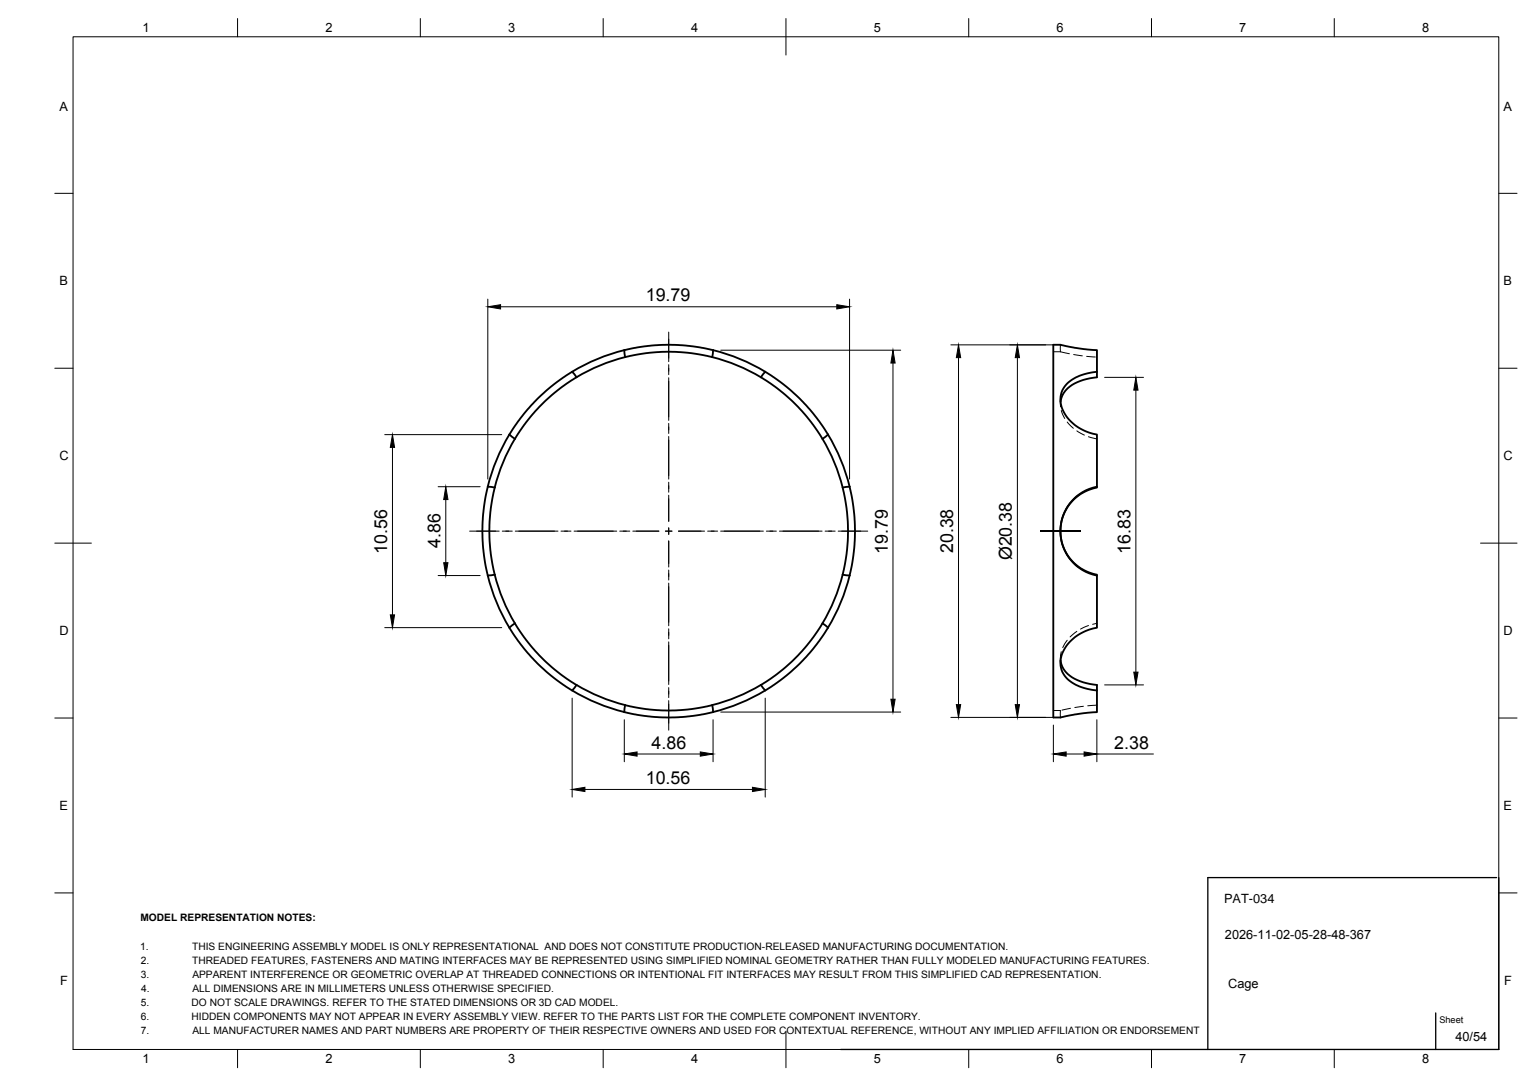
ISO-10303-21;
HEADER;
/* Generated by software containing ST-Developer
 * from STEP Tools, Inc. (www.steptools.com) 
 */

FILE_DESCRIPTION(
/* description */ ('Fatigue rig crank-slider'),
/* implementation_level */ '2;1');

FILE_NAME(
/* name */ 'Cage.step',
/* time_stamp */ '2026-10-28T03:24:50-07:00',
/* author */ (''),
/* organization */ (''),
/* preprocessor_version */ 'ST-DEVELOPER v20.2',
/* originating_system */ 'Autodesk Translation Framework v15.17.0.0',
/* authorisation */ '');

FILE_SCHEMA (('AUTOMOTIVE_DESIGN { 1 0 10303 214 3 1 1 }'));
ENDSEC;

DATA;
#10=MECHANICAL_DESIGN_GEOMETRIC_PRESENTATION_REPRESENTATION('',(#630),#16911);
#451=B_SPLINE_CURVE_WITH_KNOTS('',3,(#15536,#15537,#15538,#15539,#15540,
#15541,#15542,#15543,#15544,#15545,#15546,#15547,#15548,#15549,#15550,#15551,
#15552,#15553,#15554,#15555,#15556,#15557),.UNSPECIFIED.,.F.,.F.,(4,2,2,
2,2,2,2,2,2,2,4),(0.0473477652366656,0.126350602536658,0.189525903804987,
0.252701205073317,0.313298422430275,0.373895639787233,0.434492857144191,
0.495090074501149,0.558265375769478,0.621440677037807,0.7004435143378),
 .UNSPECIFIED.);
#452=B_SPLINE_CURVE_WITH_KNOTS('',3,(#15561,#15562,#15563,#15564,#15565,
#15566,#15567,#15568,#15569,#15570,#15571,#15572,#15573,#15574,#15575,#15576,
#15577,#15578,#15579,#15580,#15581,#15582),.UNSPECIFIED.,.F.,.F.,(4,2,2,
2,2,2,2,2,2,2,4),(0.0464897534940957,0.0852567806515119,0.170513561303024,
0.246687263103517,0.308657850341199,0.370628437578881,0.432599024816563,
0.494569612054245,0.570743313854739,0.656000094506251,0.694767121663666),
 .UNSPECIFIED.);
#453=B_SPLINE_CURVE_WITH_KNOTS('',3,(#15588,#15589,#15590,#15591,#15592,
#15593,#15594,#15595,#15596,#15597,#15598,#15599,#15600,#15601,#15602,#15603,
#15604,#15605,#15606,#15607,#15608,#15609),.UNSPECIFIED.,.F.,.F.,(4,2,2,
2,2,2,2,2,2,2,4),(0.0464897534940957,0.0852567806515118,0.170513561303024,
0.246687263103517,0.308657850341199,0.370628437578881,0.432599024816563,
0.494569612054245,0.570743313854738,0.65600009450625,0.694767121663666),
 .UNSPECIFIED.);
#454=B_SPLINE_CURVE_WITH_KNOTS('',3,(#15613,#15614,#15615,#15616,#15617,
#15618,#15619,#15620,#15621,#15622,#15623,#15624,#15625,#15626,#15627,#15628,
#15629,#15630,#15631,#15632,#15633,#15634),.UNSPECIFIED.,.F.,.F.,(4,2,2,
2,2,2,2,2,2,2,4),(0.0464897534940957,0.0852567806515119,0.170513561303024,
0.246687263103517,0.308657850341199,0.370628437578881,0.432599024816563,
0.494569612054245,0.570743313854739,0.656000094506251,0.694767121663666),
 .UNSPECIFIED.);
#455=B_SPLINE_CURVE_WITH_KNOTS('',3,(#15638,#15639,#15640,#15641,#15642,
#15643,#15644,#15645,#15646,#15647,#15648,#15649),.UNSPECIFIED.,.F.,.F.,
(4,2,2,2,2,4),(0.0464897534940957,0.0852567806515119,0.170513561303024,
0.246687263103517,0.308657850341199,0.370628437578881),.UNSPECIFIED.);
#456=B_SPLINE_CURVE_WITH_KNOTS('',3,(#15654,#15655,#15656,#15657,#15658,
#15659,#15660,#15661,#15662,#15663,#15664,#15665),.UNSPECIFIED.,.F.,.F.,
(4,2,2,2,2,4),(0.370628437578881,0.432599024816563,0.494569612054245,0.570743313854738,
0.65600009450625,0.694767121663666),.UNSPECIFIED.);
#457=B_SPLINE_CURVE_WITH_KNOTS('',3,(#15669,#15670,#15671,#15672,#15673,
#15674,#15675,#15676,#15677,#15678,#15679,#15680,#15681,#15682,#15683,#15684,
#15685,#15686,#15687,#15688,#15689,#15690),.UNSPECIFIED.,.F.,.F.,(4,2,2,
2,2,2,2,2,2,2,4),(0.0464897534940957,0.0852567806515121,0.170513561303024,
0.246687263103518,0.308657850341199,0.370628437578881,0.432599024816563,
0.494569612054245,0.570743313854738,0.65600009450625,0.694767121663666),
 .UNSPECIFIED.);
#458=B_SPLINE_CURVE_WITH_KNOTS('',3,(#15694,#15695,#15696,#15697,#15698,
#15699,#15700,#15701,#15702,#15703,#15704,#15705,#15706,#15707,#15708,#15709,
#15710,#15711,#15712,#15713,#15714,#15715),.UNSPECIFIED.,.F.,.F.,(4,2,2,
2,2,2,2,2,2,2,4),(0.0464897534940957,0.0852567806515119,0.170513561303024,
0.246687263103517,0.308657850341199,0.370628437578881,0.432599024816563,
0.494569612054245,0.570743313854738,0.65600009450625,0.694767121663667),
 .UNSPECIFIED.);
#459=B_SPLINE_CURVE_WITH_KNOTS('',3,(#15719,#15720,#15721,#15722,#15723,
#15724,#15725,#15726,#15727,#15728,#15729,#15730,#15731,#15732,#15733,#15734,
#15735,#15736,#15737,#15738,#15739,#15740),.UNSPECIFIED.,.F.,.F.,(4,2,2,
2,2,2,2,2,2,2,4),(0.0464897534940957,0.0852567806515119,0.170513561303024,
0.246687263103517,0.308657850341199,0.370628437578881,0.432599024816563,
0.494569612054245,0.570743313854738,0.65600009450625,0.694767121663666),
 .UNSPECIFIED.);
#460=B_SPLINE_CURVE_WITH_KNOTS('',3,(#15744,#15745,#15746,#15747,#15748,
#15749,#15750,#15751,#15752,#15753,#15754,#15755,#15756,#15757,#15758,#15759,
#15760,#15761,#15762,#15763,#15764,#15765),.UNSPECIFIED.,.F.,.F.,(4,2,2,
2,2,2,2,2,2,2,4),(0.0464897534940957,0.0852567806515119,0.170513561303024,
0.246687263103517,0.308657850341199,0.370628437578881,0.432599024816563,
0.494569612054245,0.570743313854739,0.656000094506251,0.694767121663667),
 .UNSPECIFIED.);
#461=B_SPLINE_CURVE_WITH_KNOTS('',3,(#15773,#15774,#15775,#15776,#15777,
#15778,#15779,#15780,#15781,#15782,#15783,#15784,#15785,#15786,#15787,#15788,
#15789,#15790,#15791,#15792,#15793,#15794),.UNSPECIFIED.,.F.,.F.,(4,2,2,
2,2,2,2,2,2,2,4),(0.0473477652366656,0.126350602536658,0.189525903804987,
0.252701205073316,0.313298422430274,0.373895639787232,0.434492857144191,
0.495090074501149,0.558265375769478,0.621440677037807,0.7004435143378),
 .UNSPECIFIED.);
#462=B_SPLINE_CURVE_WITH_KNOTS('',3,(#15802,#15803,#15804,#15805,#15806,
#15807,#15808,#15809,#15810,#15811,#15812,#15813,#15814,#15815,#15816,#15817,
#15818,#15819,#15820,#15821,#15822,#15823),.UNSPECIFIED.,.F.,.F.,(4,2,2,
2,2,2,2,2,2,2,4),(0.0473477652366656,0.126350602536658,0.189525903804987,
0.252701205073317,0.313298422430275,0.373895639787233,0.434492857144191,
0.495090074501149,0.558265375769478,0.621440677037807,0.7004435143378),
 .UNSPECIFIED.);
#463=B_SPLINE_CURVE_WITH_KNOTS('',3,(#15832,#15833,#15834,#15835,#15836,
#15837,#15838,#15839,#15840,#15841,#15842,#15843),.UNSPECIFIED.,.F.,.F.,
(4,2,2,2,2,4),(0.0473477652366656,0.126350602536658,0.189525903804987,0.252701205073316,
0.313298422430275,0.373895639787233),.UNSPECIFIED.);
#464=B_SPLINE_CURVE_WITH_KNOTS('',3,(#15845,#15846,#15847,#15848,#15849,
#15850,#15851,#15852,#15853,#15854,#15855,#15856),.UNSPECIFIED.,.F.,.F.,
(4,2,2,2,2,4),(0.373895639787233,0.434492857144191,0.495090074501149,0.558265375769478,
0.621440677037807,0.7004435143378),.UNSPECIFIED.);
#465=B_SPLINE_CURVE_WITH_KNOTS('',3,(#15863,#15864,#15865,#15866,#15867,
#15868,#15869,#15870,#15871,#15872,#15873,#15874,#15875,#15876,#15877,#15878,
#15879,#15880,#15881,#15882,#15883,#15884),.UNSPECIFIED.,.F.,.F.,(4,2,2,
2,2,2,2,2,2,2,4),(0.0473477652366656,0.126350602536658,0.189525903804987,
0.252701205073316,0.313298422430275,0.373895639787233,0.434492857144191,
0.495090074501149,0.558265375769478,0.621440677037807,0.7004435143378),
 .UNSPECIFIED.);
#466=B_SPLINE_CURVE_WITH_KNOTS('',3,(#15892,#15893,#15894,#15895,#15896,
#15897,#15898,#15899,#15900,#15901,#15902,#15903,#15904,#15905,#15906,#15907,
#15908,#15909,#15910,#15911,#15912,#15913),.UNSPECIFIED.,.F.,.F.,(4,2,2,
2,2,2,2,2,2,2,4),(0.0473477652366656,0.126350602536658,0.189525903804987,
0.252701205073317,0.313298422430275,0.373895639787233,0.434492857144191,
0.495090074501149,0.558265375769478,0.621440677037807,0.7004435143378),
 .UNSPECIFIED.);
#467=B_SPLINE_CURVE_WITH_KNOTS('',3,(#15921,#15922,#15923,#15924,#15925,
#15926,#15927,#15928,#15929,#15930,#15931,#15932,#15933,#15934,#15935,#15936,
#15937,#15938,#15939,#15940,#15941,#15942),.UNSPECIFIED.,.F.,.F.,(4,2,2,
2,2,2,2,2,2,2,4),(0.0473477652366656,0.126350602536658,0.189525903804987,
0.252701205073316,0.313298422430275,0.373895639787233,0.434492857144191,
0.495090074501149,0.558265375769478,0.621440677037807,0.7004435143378),
 .UNSPECIFIED.);
#468=B_SPLINE_CURVE_WITH_KNOTS('',3,(#15951,#15952,#15953,#15954,#15955,
#15956,#15957,#15958,#15959,#15960,#15961,#15962,#15963,#15964,#15965,#15966,
#15967,#15968,#15969,#15970,#15971,#15972),.UNSPECIFIED.,.F.,.F.,(4,2,2,
2,2,2,2,2,2,2,4),(0.0473477652366656,0.126350602536658,0.189525903804987,
0.252701205073317,0.313298422430275,0.373895639787233,0.434492857144191,
0.495090074501149,0.558265375769478,0.621440677037807,0.7004435143378),
 .UNSPECIFIED.);
#479=SPHERICAL_SURFACE('',#10165,0.247676);
#480=SPHERICAL_SURFACE('',#10181,0.247676);
#481=SPHERICAL_SURFACE('',#10186,0.247676);
#482=SPHERICAL_SURFACE('',#10191,0.247676);
#483=SPHERICAL_SURFACE('',#10196,0.247676);
#484=SPHERICAL_SURFACE('',#10201,0.247676);
#485=SPHERICAL_SURFACE('',#10206,0.247676);
#486=SPHERICAL_SURFACE('',#10214,0.247676);
#522=SHAPE_REPRESENTATION_RELATIONSHIP('SRR','None',#17165,#572);
#572=ADVANCED_BREP_SHAPE_REPRESENTATION('',(#687),#16894);
#630=STYLED_ITEM('',(#17487),#687);
#687=MANIFOLD_SOLID_BREP('Continuous crown cage',#8923);
#858=FACE_BOUND('',#2265,.T.);
#1098=PLANE('',#10178);
#1099=PLANE('',#10183);
#1100=PLANE('',#10188);
#1101=PLANE('',#10193);
#1102=PLANE('',#10198);
#1103=PLANE('',#10203);
#1104=PLANE('',#10212);
#1105=PLANE('',#10216);
#1106=PLANE('',#10217);
#1566=FACE_OUTER_BOUND('',#2247,.T.);
#1567=FACE_OUTER_BOUND('',#2248,.T.);
#1568=FACE_OUTER_BOUND('',#2249,.T.);
#1569=FACE_OUTER_BOUND('',#2250,.T.);
#1570=FACE_OUTER_BOUND('',#2251,.T.);
#1571=FACE_OUTER_BOUND('',#2252,.T.);
#1572=FACE_OUTER_BOUND('',#2253,.T.);
#1573=FACE_OUTER_BOUND('',#2254,.T.);
#1574=FACE_OUTER_BOUND('',#2255,.T.);
#1575=FACE_OUTER_BOUND('',#2256,.T.);
#1576=FACE_OUTER_BOUND('',#2257,.T.);
#1577=FACE_OUTER_BOUND('',#2258,.T.);
#1578=FACE_OUTER_BOUND('',#2259,.T.);
#1579=FACE_OUTER_BOUND('',#2260,.T.);
#1580=FACE_OUTER_BOUND('',#2261,.T.);
#1581=FACE_OUTER_BOUND('',#2262,.T.);
#1582=FACE_OUTER_BOUND('',#2263,.T.);
#1583=FACE_OUTER_BOUND('',#2264,.T.);
#1584=FACE_OUTER_BOUND('',#2266,.T.);
#2247=EDGE_LOOP('',(#7420,#7421,#7422,#7423));
#2248=EDGE_LOOP('',(#7424,#7425,#7426,#7427,#7428,#7429,#7430,#7431,#7432,
#7433,#7434,#7435,#7436,#7437,#7438,#7439,#7440,#7441,#7442,#7443));
#2249=EDGE_LOOP('',(#7444,#7445,#7446,#7447));
#2250=EDGE_LOOP('',(#7448,#7449,#7450,#7451));
#2251=EDGE_LOOP('',(#7452,#7453,#7454,#7455));
#2252=EDGE_LOOP('',(#7456,#7457,#7458,#7459));
#2253=EDGE_LOOP('',(#7460,#7461,#7462,#7463));
#2254=EDGE_LOOP('',(#7464,#7465,#7466,#7467,#7468,#7469));
#2255=EDGE_LOOP('',(#7470,#7471,#7472,#7473));
#2256=EDGE_LOOP('',(#7474,#7475,#7476,#7477));
#2257=EDGE_LOOP('',(#7478,#7479,#7480,#7481));
#2258=EDGE_LOOP('',(#7482,#7483,#7484,#7485));
#2259=EDGE_LOOP('',(#7486,#7487,#7488,#7489));
#2260=EDGE_LOOP('',(#7490,#7491,#7492,#7493));
#2261=EDGE_LOOP('',(#7494,#7495,#7496,#7497,#7498,#7499,#7500,#7501,#7502,
#7503,#7504,#7505,#7506,#7507,#7508,#7509,#7510,#7511,#7512,#7513));
#2262=EDGE_LOOP('',(#7514,#7515,#7516,#7517));
#2263=EDGE_LOOP('',(#7518,#7519,#7520,#7521));
#2264=EDGE_LOOP('',(#7522));
#2265=EDGE_LOOP('',(#7523));
#2266=EDGE_LOOP('',(#7524,#7525,#7526,#7527));
#2857=LINE('',#15651,#3503);
#2858=LINE('',#15947,#3504);
#3503=VECTOR('',#12321,1.019052);
#3504=VECTOR('',#12398,0.980948);
#4031=CIRCLE('',#10166,0.243053047864041);
#4032=CIRCLE('',#10167,0.243053047864041);
#4033=CIRCLE('',#10169,1.019052);
#4034=CIRCLE('',#10170,1.019052);
#4035=CIRCLE('',#10171,1.019052);
#4036=CIRCLE('',#10172,1.019052);
#4037=CIRCLE('',#10173,1.019052);
#4038=CIRCLE('',#10174,1.019052);
#4039=CIRCLE('',#10175,1.019052);
#4040=CIRCLE('',#10176,1.019052);
#4041=CIRCLE('',#10177,1.019052);
#4042=CIRCLE('',#10179,0.980948);
#4043=CIRCLE('',#10180,0.243053047864041);
#4044=CIRCLE('',#10182,0.243053047864041);
#4045=CIRCLE('',#10184,0.980948);
#4046=CIRCLE('',#10185,0.243053047864041);
#4047=CIRCLE('',#10187,0.243053047864041);
#4048=CIRCLE('',#10189,0.980948);
#4049=CIRCLE('',#10190,0.243053047864041);
#4050=CIRCLE('',#10192,0.243053047864041);
#4051=CIRCLE('',#10194,0.980948);
#4052=CIRCLE('',#10195,0.243053047864041);
#4053=CIRCLE('',#10197,0.243053047864041);
#4054=CIRCLE('',#10199,0.980948);
#4055=CIRCLE('',#10200,0.243053047864041);
#4056=CIRCLE('',#10202,0.243053047864041);
#4057=CIRCLE('',#10204,0.980948);
#4058=CIRCLE('',#10205,0.243053047864041);
#4059=CIRCLE('',#10207,0.243053047864041);
#4060=CIRCLE('',#10209,0.980948);
#4061=CIRCLE('',#10210,0.980948);
#4062=CIRCLE('',#10211,0.980948);
#4063=CIRCLE('',#10213,0.243053047864041);
#4064=CIRCLE('',#10215,0.243053047864041);
#4641=VERTEX_POINT('',#15534);
#4642=VERTEX_POINT('',#15535);
#4643=VERTEX_POINT('',#15558);
#4644=VERTEX_POINT('',#15560);
#4645=VERTEX_POINT('',#15585);
#4646=VERTEX_POINT('',#15587);
#4647=VERTEX_POINT('',#15610);
#4648=VERTEX_POINT('',#15612);
#4649=VERTEX_POINT('',#15635);
#4650=VERTEX_POINT('',#15637);
#4651=VERTEX_POINT('',#15650);
#4652=VERTEX_POINT('',#15653);
#4653=VERTEX_POINT('',#15666);
#4654=VERTEX_POINT('',#15668);
#4655=VERTEX_POINT('',#15691);
#4656=VERTEX_POINT('',#15693);
#4657=VERTEX_POINT('',#15716);
#4658=VERTEX_POINT('',#15718);
#4659=VERTEX_POINT('',#15741);
#4660=VERTEX_POINT('',#15743);
#4661=VERTEX_POINT('',#15768);
#4662=VERTEX_POINT('',#15772);
#4663=VERTEX_POINT('',#15797);
#4664=VERTEX_POINT('',#15801);
#4665=VERTEX_POINT('',#15826);
#4666=VERTEX_POINT('',#15830);
#4667=VERTEX_POINT('',#15831);
#4668=VERTEX_POINT('',#15858);
#4669=VERTEX_POINT('',#15862);
#4670=VERTEX_POINT('',#15887);
#4671=VERTEX_POINT('',#15891);
#4672=VERTEX_POINT('',#15916);
#4673=VERTEX_POINT('',#15920);
#4674=VERTEX_POINT('',#15945);
#4675=VERTEX_POINT('',#15948);
#4676=VERTEX_POINT('',#15950);
#5608=EDGE_CURVE('',#4641,#4642,#451,.T.);
#5609=EDGE_CURVE('',#4643,#4641,#4031,.T.);
#5610=EDGE_CURVE('',#4644,#4643,#452,.T.);
#5611=EDGE_CURVE('',#4642,#4644,#4032,.T.);
#5612=EDGE_CURVE('',#4645,#4643,#4033,.T.);
#5613=EDGE_CURVE('',#4645,#4646,#453,.T.);
#5614=EDGE_CURVE('',#4647,#4646,#4034,.T.);
#5615=EDGE_CURVE('',#4647,#4648,#454,.T.);
#5616=EDGE_CURVE('',#4649,#4648,#4035,.T.);
#5617=EDGE_CURVE('',#4649,#4650,#455,.T.);
#5618=EDGE_CURVE('',#4650,#4651,#2857,.T.);
#5619=EDGE_CURVE('',#4651,#4651,#4036,.T.);
#5620=EDGE_CURVE('',#4650,#4652,#456,.T.);
#5621=EDGE_CURVE('',#4653,#4652,#4037,.T.);
#5622=EDGE_CURVE('',#4653,#4654,#457,.T.);
#5623=EDGE_CURVE('',#4655,#4654,#4038,.T.);
#5624=EDGE_CURVE('',#4655,#4656,#458,.T.);
#5625=EDGE_CURVE('',#4657,#4656,#4039,.T.);
#5626=EDGE_CURVE('',#4657,#4658,#459,.T.);
#5627=EDGE_CURVE('',#4659,#4658,#4040,.T.);
#5628=EDGE_CURVE('',#4659,#4660,#460,.T.);
#5629=EDGE_CURVE('',#4644,#4660,#4041,.T.);
#5630=EDGE_CURVE('',#4641,#4661,#4042,.T.);
#5631=EDGE_CURVE('',#4661,#4645,#4043,.T.);
#5632=EDGE_CURVE('',#4662,#4661,#461,.T.);
#5633=EDGE_CURVE('',#4646,#4662,#4044,.T.);
#5634=EDGE_CURVE('',#4662,#4663,#4045,.T.);
#5635=EDGE_CURVE('',#4663,#4647,#4046,.T.);
#5636=EDGE_CURVE('',#4664,#4663,#462,.T.);
#5637=EDGE_CURVE('',#4648,#4664,#4047,.T.);
#5638=EDGE_CURVE('',#4664,#4665,#4048,.T.);
#5639=EDGE_CURVE('',#4665,#4649,#4049,.T.);
#5640=EDGE_CURVE('',#4666,#4667,#463,.T.);
#5641=EDGE_CURVE('',#4652,#4666,#4050,.T.);
#5642=EDGE_CURVE('',#4667,#4665,#464,.T.);
#5643=EDGE_CURVE('',#4666,#4668,#4051,.T.);
#5644=EDGE_CURVE('',#4668,#4653,#4052,.T.);
#5645=EDGE_CURVE('',#4669,#4668,#465,.T.);
#5646=EDGE_CURVE('',#4654,#4669,#4053,.T.);
#5647=EDGE_CURVE('',#4669,#4670,#4054,.T.);
#5648=EDGE_CURVE('',#4670,#4655,#4055,.T.);
#5649=EDGE_CURVE('',#4671,#4670,#466,.T.);
#5650=EDGE_CURVE('',#4656,#4671,#4056,.T.);
#5651=EDGE_CURVE('',#4671,#4672,#4057,.T.);
#5652=EDGE_CURVE('',#4672,#4657,#4058,.T.);
#5653=EDGE_CURVE('',#4673,#4672,#467,.T.);
#5654=EDGE_CURVE('',#4658,#4673,#4059,.T.);
#5655=EDGE_CURVE('',#4674,#4674,#4060,.T.);
#5656=EDGE_CURVE('',#4674,#4667,#2858,.T.);
#5657=EDGE_CURVE('',#4675,#4642,#4061,.T.);
#5658=EDGE_CURVE('',#4675,#4676,#468,.T.);
#5659=EDGE_CURVE('',#4673,#4676,#4062,.T.);
#5660=EDGE_CURVE('',#4660,#4675,#4063,.T.);
#5661=EDGE_CURVE('',#4676,#4659,#4064,.T.);
#7420=ORIENTED_EDGE('',*,*,#5608,.F.);
#7421=ORIENTED_EDGE('',*,*,#5609,.F.);
#7422=ORIENTED_EDGE('',*,*,#5610,.F.);
#7423=ORIENTED_EDGE('',*,*,#5611,.F.);
#7424=ORIENTED_EDGE('',*,*,#5610,.T.);
#7425=ORIENTED_EDGE('',*,*,#5612,.F.);
#7426=ORIENTED_EDGE('',*,*,#5613,.T.);
#7427=ORIENTED_EDGE('',*,*,#5614,.F.);
#7428=ORIENTED_EDGE('',*,*,#5615,.T.);
#7429=ORIENTED_EDGE('',*,*,#5616,.F.);
#7430=ORIENTED_EDGE('',*,*,#5617,.T.);
#7431=ORIENTED_EDGE('',*,*,#5618,.T.);
#7432=ORIENTED_EDGE('',*,*,#5619,.F.);
#7433=ORIENTED_EDGE('',*,*,#5618,.F.);
#7434=ORIENTED_EDGE('',*,*,#5620,.T.);
#7435=ORIENTED_EDGE('',*,*,#5621,.F.);
#7436=ORIENTED_EDGE('',*,*,#5622,.T.);
#7437=ORIENTED_EDGE('',*,*,#5623,.F.);
#7438=ORIENTED_EDGE('',*,*,#5624,.T.);
#7439=ORIENTED_EDGE('',*,*,#5625,.F.);
#7440=ORIENTED_EDGE('',*,*,#5626,.T.);
#7441=ORIENTED_EDGE('',*,*,#5627,.F.);
#7442=ORIENTED_EDGE('',*,*,#5628,.T.);
#7443=ORIENTED_EDGE('',*,*,#5629,.F.);
#7444=ORIENTED_EDGE('',*,*,#5609,.T.);
#7445=ORIENTED_EDGE('',*,*,#5630,.T.);
#7446=ORIENTED_EDGE('',*,*,#5631,.T.);
#7447=ORIENTED_EDGE('',*,*,#5612,.T.);
#7448=ORIENTED_EDGE('',*,*,#5632,.F.);
#7449=ORIENTED_EDGE('',*,*,#5633,.F.);
#7450=ORIENTED_EDGE('',*,*,#5613,.F.);
#7451=ORIENTED_EDGE('',*,*,#5631,.F.);
#7452=ORIENTED_EDGE('',*,*,#5633,.T.);
#7453=ORIENTED_EDGE('',*,*,#5634,.T.);
#7454=ORIENTED_EDGE('',*,*,#5635,.T.);
#7455=ORIENTED_EDGE('',*,*,#5614,.T.);
#7456=ORIENTED_EDGE('',*,*,#5636,.F.);
#7457=ORIENTED_EDGE('',*,*,#5637,.F.);
#7458=ORIENTED_EDGE('',*,*,#5615,.F.);
#7459=ORIENTED_EDGE('',*,*,#5635,.F.);
#7460=ORIENTED_EDGE('',*,*,#5637,.T.);
#7461=ORIENTED_EDGE('',*,*,#5638,.T.);
#7462=ORIENTED_EDGE('',*,*,#5639,.T.);
#7463=ORIENTED_EDGE('',*,*,#5616,.T.);
#7464=ORIENTED_EDGE('',*,*,#5640,.F.);
#7465=ORIENTED_EDGE('',*,*,#5641,.F.);
#7466=ORIENTED_EDGE('',*,*,#5620,.F.);
#7467=ORIENTED_EDGE('',*,*,#5617,.F.);
#7468=ORIENTED_EDGE('',*,*,#5639,.F.);
#7469=ORIENTED_EDGE('',*,*,#5642,.F.);
#7470=ORIENTED_EDGE('',*,*,#5641,.T.);
#7471=ORIENTED_EDGE('',*,*,#5643,.T.);
#7472=ORIENTED_EDGE('',*,*,#5644,.T.);
#7473=ORIENTED_EDGE('',*,*,#5621,.T.);
#7474=ORIENTED_EDGE('',*,*,#5645,.F.);
#7475=ORIENTED_EDGE('',*,*,#5646,.F.);
#7476=ORIENTED_EDGE('',*,*,#5622,.F.);
#7477=ORIENTED_EDGE('',*,*,#5644,.F.);
#7478=ORIENTED_EDGE('',*,*,#5646,.T.);
#7479=ORIENTED_EDGE('',*,*,#5647,.T.);
#7480=ORIENTED_EDGE('',*,*,#5648,.T.);
#7481=ORIENTED_EDGE('',*,*,#5623,.T.);
#7482=ORIENTED_EDGE('',*,*,#5649,.F.);
#7483=ORIENTED_EDGE('',*,*,#5650,.F.);
#7484=ORIENTED_EDGE('',*,*,#5624,.F.);
#7485=ORIENTED_EDGE('',*,*,#5648,.F.);
#7486=ORIENTED_EDGE('',*,*,#5650,.T.);
#7487=ORIENTED_EDGE('',*,*,#5651,.T.);
#7488=ORIENTED_EDGE('',*,*,#5652,.T.);
#7489=ORIENTED_EDGE('',*,*,#5625,.T.);
#7490=ORIENTED_EDGE('',*,*,#5626,.F.);
#7491=ORIENTED_EDGE('',*,*,#5652,.F.);
#7492=ORIENTED_EDGE('',*,*,#5653,.F.);
#7493=ORIENTED_EDGE('',*,*,#5654,.F.);
#7494=ORIENTED_EDGE('',*,*,#5655,.F.);
#7495=ORIENTED_EDGE('',*,*,#5656,.T.);
#7496=ORIENTED_EDGE('',*,*,#5642,.T.);
#7497=ORIENTED_EDGE('',*,*,#5638,.F.);
#7498=ORIENTED_EDGE('',*,*,#5636,.T.);
#7499=ORIENTED_EDGE('',*,*,#5634,.F.);
#7500=ORIENTED_EDGE('',*,*,#5632,.T.);
#7501=ORIENTED_EDGE('',*,*,#5630,.F.);
#7502=ORIENTED_EDGE('',*,*,#5608,.T.);
#7503=ORIENTED_EDGE('',*,*,#5657,.F.);
#7504=ORIENTED_EDGE('',*,*,#5658,.T.);
#7505=ORIENTED_EDGE('',*,*,#5659,.F.);
#7506=ORIENTED_EDGE('',*,*,#5653,.T.);
#7507=ORIENTED_EDGE('',*,*,#5651,.F.);
#7508=ORIENTED_EDGE('',*,*,#5649,.T.);
#7509=ORIENTED_EDGE('',*,*,#5647,.F.);
#7510=ORIENTED_EDGE('',*,*,#5645,.T.);
#7511=ORIENTED_EDGE('',*,*,#5643,.F.);
#7512=ORIENTED_EDGE('',*,*,#5640,.T.);
#7513=ORIENTED_EDGE('',*,*,#5656,.F.);
#7514=ORIENTED_EDGE('',*,*,#5611,.T.);
#7515=ORIENTED_EDGE('',*,*,#5629,.T.);
#7516=ORIENTED_EDGE('',*,*,#5660,.T.);
#7517=ORIENTED_EDGE('',*,*,#5657,.T.);
#7518=ORIENTED_EDGE('',*,*,#5628,.F.);
#7519=ORIENTED_EDGE('',*,*,#5661,.F.);
#7520=ORIENTED_EDGE('',*,*,#5658,.F.);
#7521=ORIENTED_EDGE('',*,*,#5660,.F.);
#7522=ORIENTED_EDGE('',*,*,#5619,.T.);
#7523=ORIENTED_EDGE('',*,*,#5655,.T.);
#7524=ORIENTED_EDGE('',*,*,#5654,.T.);
#7525=ORIENTED_EDGE('',*,*,#5659,.T.);
#7526=ORIENTED_EDGE('',*,*,#5661,.T.);
#7527=ORIENTED_EDGE('',*,*,#5627,.T.);
#8319=CYLINDRICAL_SURFACE('',#10168,1.019052);
#8320=CYLINDRICAL_SURFACE('',#10208,0.980948);
#8704=ADVANCED_FACE('',(#1566),#479,.F.);
#8705=ADVANCED_FACE('',(#1567),#8319,.T.);
#8706=ADVANCED_FACE('',(#1568),#1098,.T.);
#8707=ADVANCED_FACE('',(#1569),#480,.F.);
#8708=ADVANCED_FACE('',(#1570),#1099,.T.);
#8709=ADVANCED_FACE('',(#1571),#481,.F.);
#8710=ADVANCED_FACE('',(#1572),#1100,.T.);
#8711=ADVANCED_FACE('',(#1573),#482,.F.);
#8712=ADVANCED_FACE('',(#1574),#1101,.T.);
#8713=ADVANCED_FACE('',(#1575),#483,.F.);
#8714=ADVANCED_FACE('',(#1576),#1102,.T.);
#8715=ADVANCED_FACE('',(#1577),#484,.F.);
#8716=ADVANCED_FACE('',(#1578),#1103,.T.);
#8717=ADVANCED_FACE('',(#1579),#485,.F.);
#8718=ADVANCED_FACE('',(#1580),#8320,.F.);
#8719=ADVANCED_FACE('',(#1581),#1104,.T.);
#8720=ADVANCED_FACE('',(#1582),#486,.F.);
#8721=ADVANCED_FACE('',(#1583,#858),#1105,.T.);
#8722=ADVANCED_FACE('',(#1584),#1106,.T.);
#8923=CLOSED_SHELL('',(#8704,#8705,#8706,#8707,#8708,#8709,#8710,#8711,
#8712,#8713,#8714,#8715,#8716,#8717,#8718,#8719,#8720,#8721,#8722));
#10164=AXIS2_PLACEMENT_3D('',#15532,#12305,#12306);
#10165=AXIS2_PLACEMENT_3D('',#15533,#12307,#12308);
#10166=AXIS2_PLACEMENT_3D('',#15559,#12309,#12310);
#10167=AXIS2_PLACEMENT_3D('',#15583,#12311,#12312);
#10168=AXIS2_PLACEMENT_3D('',#15584,#12313,#12314);
#10169=AXIS2_PLACEMENT_3D('',#15586,#12315,#12316);
#10170=AXIS2_PLACEMENT_3D('',#15611,#12317,#12318);
#10171=AXIS2_PLACEMENT_3D('',#15636,#12319,#12320);
#10172=AXIS2_PLACEMENT_3D('',#15652,#12322,#12323);
#10173=AXIS2_PLACEMENT_3D('',#15667,#12324,#12325);
#10174=AXIS2_PLACEMENT_3D('',#15692,#12326,#12327);
#10175=AXIS2_PLACEMENT_3D('',#15717,#12328,#12329);
#10176=AXIS2_PLACEMENT_3D('',#15742,#12330,#12331);
#10177=AXIS2_PLACEMENT_3D('',#15766,#12332,#12333);
#10178=AXIS2_PLACEMENT_3D('',#15767,#12334,#12335);
#10179=AXIS2_PLACEMENT_3D('',#15769,#12336,#12337);
#10180=AXIS2_PLACEMENT_3D('',#15770,#12338,#12339);
#10181=AXIS2_PLACEMENT_3D('',#15771,#12340,#12341);
#10182=AXIS2_PLACEMENT_3D('',#15795,#12342,#12343);
#10183=AXIS2_PLACEMENT_3D('',#15796,#12344,#12345);
#10184=AXIS2_PLACEMENT_3D('',#15798,#12346,#12347);
#10185=AXIS2_PLACEMENT_3D('',#15799,#12348,#12349);
#10186=AXIS2_PLACEMENT_3D('',#15800,#12350,#12351);
#10187=AXIS2_PLACEMENT_3D('',#15824,#12352,#12353);
#10188=AXIS2_PLACEMENT_3D('',#15825,#12354,#12355);
#10189=AXIS2_PLACEMENT_3D('',#15827,#12356,#12357);
#10190=AXIS2_PLACEMENT_3D('',#15828,#12358,#12359);
#10191=AXIS2_PLACEMENT_3D('',#15829,#12360,#12361);
#10192=AXIS2_PLACEMENT_3D('',#15844,#12362,#12363);
#10193=AXIS2_PLACEMENT_3D('',#15857,#12364,#12365);
#10194=AXIS2_PLACEMENT_3D('',#15859,#12366,#12367);
#10195=AXIS2_PLACEMENT_3D('',#15860,#12368,#12369);
#10196=AXIS2_PLACEMENT_3D('',#15861,#12370,#12371);
#10197=AXIS2_PLACEMENT_3D('',#15885,#12372,#12373);
#10198=AXIS2_PLACEMENT_3D('',#15886,#12374,#12375);
#10199=AXIS2_PLACEMENT_3D('',#15888,#12376,#12377);
#10200=AXIS2_PLACEMENT_3D('',#15889,#12378,#12379);
#10201=AXIS2_PLACEMENT_3D('',#15890,#12380,#12381);
#10202=AXIS2_PLACEMENT_3D('',#15914,#12382,#12383);
#10203=AXIS2_PLACEMENT_3D('',#15915,#12384,#12385);
#10204=AXIS2_PLACEMENT_3D('',#15917,#12386,#12387);
#10205=AXIS2_PLACEMENT_3D('',#15918,#12388,#12389);
#10206=AXIS2_PLACEMENT_3D('',#15919,#12390,#12391);
#10207=AXIS2_PLACEMENT_3D('',#15943,#12392,#12393);
#10208=AXIS2_PLACEMENT_3D('',#15944,#12394,#12395);
#10209=AXIS2_PLACEMENT_3D('',#15946,#12396,#12397);
#10210=AXIS2_PLACEMENT_3D('',#15949,#12399,#12400);
#10211=AXIS2_PLACEMENT_3D('',#15973,#12401,#12402);
#10212=AXIS2_PLACEMENT_3D('',#15974,#12403,#12404);
#10213=AXIS2_PLACEMENT_3D('',#15975,#12405,#12406);
#10214=AXIS2_PLACEMENT_3D('',#15976,#12407,#12408);
#10215=AXIS2_PLACEMENT_3D('',#15977,#12409,#12410);
#10216=AXIS2_PLACEMENT_3D('',#15978,#12411,#12412);
#10217=AXIS2_PLACEMENT_3D('',#15979,#12413,#12414);
#12305=DIRECTION('axis',(0.,0.,1.));
#12306=DIRECTION('refdir',(1.,0.,0.));
#12307=DIRECTION('center_axis',(0.,0.,1.));
#12308=DIRECTION('ref_axis',(1.,0.,0.));
#12309=DIRECTION('center_axis',(0.,-1.,0.));
#12310=DIRECTION('ref_axis',(0.,0.,-1.));
#12311=DIRECTION('center_axis',(0.,-1.,0.));
#12312=DIRECTION('ref_axis',(0.,0.,-1.));
#12313=DIRECTION('center_axis',(0.,1.,0.));
#12314=DIRECTION('ref_axis',(1.,0.,0.));
#12315=DIRECTION('center_axis',(0.,1.,0.));
#12316=DIRECTION('ref_axis',(1.,0.,0.));
#12317=DIRECTION('center_axis',(0.,1.,0.));
#12318=DIRECTION('ref_axis',(1.,0.,0.));
#12319=DIRECTION('center_axis',(0.,1.,0.));
#12320=DIRECTION('ref_axis',(1.,0.,0.));
#12321=DIRECTION('',(0.,-1.,0.));
#12322=DIRECTION('center_axis',(0.,-1.,0.));
#12323=DIRECTION('ref_axis',(1.,0.,0.));
#12324=DIRECTION('center_axis',(0.,1.,0.));
#12325=DIRECTION('ref_axis',(1.,0.,0.));
#12326=DIRECTION('center_axis',(0.,1.,0.));
#12327=DIRECTION('ref_axis',(1.,0.,0.));
#12328=DIRECTION('center_axis',(0.,1.,0.));
#12329=DIRECTION('ref_axis',(1.,0.,0.));
#12330=DIRECTION('center_axis',(0.,1.,0.));
#12331=DIRECTION('ref_axis',(1.,0.,0.));
#12332=DIRECTION('center_axis',(0.,1.,0.));
#12333=DIRECTION('ref_axis',(1.,0.,0.));
#12334=DIRECTION('center_axis',(0.,1.,0.));
#12335=DIRECTION('ref_axis',(1.,0.,0.));
#12336=DIRECTION('center_axis',(0.,-1.,0.));
#12337=DIRECTION('ref_axis',(1.,0.,0.));
#12338=DIRECTION('center_axis',(0.,-1.,0.));
#12339=DIRECTION('ref_axis',(0.,0.,-1.));
#12340=DIRECTION('center_axis',(6.12323399573677E-17,0.,1.));
#12341=DIRECTION('ref_axis',(1.,0.,0.));
#12342=DIRECTION('center_axis',(0.,-1.,0.));
#12343=DIRECTION('ref_axis',(0.,0.,-1.));
#12344=DIRECTION('center_axis',(0.,1.,0.));
#12345=DIRECTION('ref_axis',(1.,0.,0.));
#12346=DIRECTION('center_axis',(0.,-1.,0.));
#12347=DIRECTION('ref_axis',(1.,0.,0.));
#12348=DIRECTION('center_axis',(0.,-1.,0.));
#12349=DIRECTION('ref_axis',(0.,0.,-1.));
#12350=DIRECTION('center_axis',(0.,0.,1.));
#12351=DIRECTION('ref_axis',(1.,0.,0.));
#12352=DIRECTION('center_axis',(0.,-1.,0.));
#12353=DIRECTION('ref_axis',(0.,0.,-1.));
#12354=DIRECTION('center_axis',(0.,1.,0.));
#12355=DIRECTION('ref_axis',(1.,0.,0.));
#12356=DIRECTION('center_axis',(0.,-1.,0.));
#12357=DIRECTION('ref_axis',(1.,0.,0.));
#12358=DIRECTION('center_axis',(0.,-1.,0.));
#12359=DIRECTION('ref_axis',(0.,0.,-1.));
#12360=DIRECTION('center_axis',(0.,0.,1.));
#12361=DIRECTION('ref_axis',(1.,0.,0.));
#12362=DIRECTION('center_axis',(0.,-1.,0.));
#12363=DIRECTION('ref_axis',(0.,0.,-1.));
#12364=DIRECTION('center_axis',(0.,1.,0.));
#12365=DIRECTION('ref_axis',(1.,0.,0.));
#12366=DIRECTION('center_axis',(0.,-1.,0.));
#12367=DIRECTION('ref_axis',(1.,0.,0.));
#12368=DIRECTION('center_axis',(0.,-1.,0.));
#12369=DIRECTION('ref_axis',(0.,0.,-1.));
#12370=DIRECTION('center_axis',(0.,0.,1.));
#12371=DIRECTION('ref_axis',(1.,0.,0.));
#12372=DIRECTION('center_axis',(0.,-1.,0.));
#12373=DIRECTION('ref_axis',(0.,0.,-1.));
#12374=DIRECTION('center_axis',(0.,1.,0.));
#12375=DIRECTION('ref_axis',(1.,0.,0.));
#12376=DIRECTION('center_axis',(0.,-1.,0.));
#12377=DIRECTION('ref_axis',(1.,0.,0.));
#12378=DIRECTION('center_axis',(0.,-1.,0.));
#12379=DIRECTION('ref_axis',(0.,0.,-1.));
#12380=DIRECTION('center_axis',(6.12323399573676E-17,0.,1.));
#12381=DIRECTION('ref_axis',(1.,0.,0.));
#12382=DIRECTION('center_axis',(0.,-1.,0.));
#12383=DIRECTION('ref_axis',(0.,0.,-1.));
#12384=DIRECTION('center_axis',(0.,1.,0.));
#12385=DIRECTION('ref_axis',(1.,0.,0.));
#12386=DIRECTION('center_axis',(0.,-1.,0.));
#12387=DIRECTION('ref_axis',(1.,0.,0.));
#12388=DIRECTION('center_axis',(0.,-1.,0.));
#12389=DIRECTION('ref_axis',(0.,0.,-1.));
#12390=DIRECTION('center_axis',(0.,0.,1.));
#12391=DIRECTION('ref_axis',(1.,0.,0.));
#12392=DIRECTION('center_axis',(0.,-1.,0.));
#12393=DIRECTION('ref_axis',(0.,0.,-1.));
#12394=DIRECTION('center_axis',(0.,1.,0.));
#12395=DIRECTION('ref_axis',(1.,0.,0.));
#12396=DIRECTION('center_axis',(0.,1.,0.));
#12397=DIRECTION('ref_axis',(1.,0.,0.));
#12398=DIRECTION('',(0.,1.,0.));
#12399=DIRECTION('center_axis',(0.,-1.,0.));
#12400=DIRECTION('ref_axis',(1.,0.,0.));
#12401=DIRECTION('center_axis',(0.,-1.,0.));
#12402=DIRECTION('ref_axis',(1.,0.,0.));
#12403=DIRECTION('center_axis',(0.,1.,0.));
#12404=DIRECTION('ref_axis',(1.,0.,0.));
#12405=DIRECTION('center_axis',(0.,-1.,0.));
#12406=DIRECTION('ref_axis',(0.,0.,-1.));
#12407=DIRECTION('center_axis',(0.,0.,1.));
#12408=DIRECTION('ref_axis',(1.,0.,0.));
#12409=DIRECTION('center_axis',(0.,-1.,0.));
#12410=DIRECTION('ref_axis',(0.,0.,-1.));
#12411=DIRECTION('center_axis',(0.,-1.,0.));
#12412=DIRECTION('ref_axis',(-1.,0.,0.));
#12413=DIRECTION('center_axis',(0.,1.,0.));
#12414=DIRECTION('ref_axis',(1.,0.,0.));
#15532=CARTESIAN_POINT('',(0.,0.,0.));
#15533=CARTESIAN_POINT('Origin',(0.707106781186547,0.,0.707106781186548));
#15534=CARTESIAN_POINT('',(0.504455939115715,-0.04763,0.841298510752802));
#15535=CARTESIAN_POINT('',(0.841298510752802,-0.04763,0.504455939115715));
#15536=CARTESIAN_POINT('Ctrl Pts',(0.504455939115715,-0.04763,0.841298510752802));
#15537=CARTESIAN_POINT('Ctrl Pts',(0.508899795931835,-0.0740444353928835,
0.838633903678357));
#15538=CARTESIAN_POINT('Ctrl Pts',(0.517157748491652,-0.0999305678883309,
0.833661031856294));
#15539=CARTESIAN_POINT('Ctrl Pts',(0.537715343527944,-0.142345102874864,
0.820511285096538));
#15540=CARTESIAN_POINT('Ctrl Pts',(0.548874290046456,-0.159766064500479,
0.813159949759));
#15541=CARTESIAN_POINT('Ctrl Pts',(0.573915184558107,-0.190326085855194,
0.795684265985089));
#15542=CARTESIAN_POINT('Ctrl Pts',(0.587792702767295,-0.203463743702801,
0.78555112003688));
#15543=CARTESIAN_POINT('Ctrl Pts',(0.615966552324775,-0.224161999508995,
0.763642258217233));
#15544=CARTESIAN_POINT('Ctrl Pts',(0.631684198665438,-0.232861760990032,
0.750785745543687));
#15545=CARTESIAN_POINT('Ctrl Pts',(0.663382628119203,-0.244251601209411,
0.722929908501543));
#15546=CARTESIAN_POINT('Ctrl Pts',(0.679352081686668,-0.246942143572133,
0.707917883896095));
#15547=CARTESIAN_POINT('Ctrl Pts',(0.707917883896095,-0.246942143572133,
0.679352081686668));
#15548=CARTESIAN_POINT('Ctrl Pts',(0.722929908501543,-0.244251601209411,
0.663382628119203));
#15549=CARTESIAN_POINT('Ctrl Pts',(0.750785745543687,-0.232861760990032,
0.631684198665439));
#15550=CARTESIAN_POINT('Ctrl Pts',(0.763642258217232,-0.224161999508995,
0.615966552324775));
#15551=CARTESIAN_POINT('Ctrl Pts',(0.78555112003688,-0.203463743702801,
0.587792702767295));
#15552=CARTESIAN_POINT('Ctrl Pts',(0.795684265985088,-0.190326085855194,
0.573915184558108));
#15553=CARTESIAN_POINT('Ctrl Pts',(0.813159949759,-0.15976606450048,0.548874290046456));
#15554=CARTESIAN_POINT('Ctrl Pts',(0.820511285096538,-0.142345102874864,
0.537715343527944));
#15555=CARTESIAN_POINT('Ctrl Pts',(0.833661031856294,-0.099930567888331,
0.517157748491653));
#15556=CARTESIAN_POINT('Ctrl Pts',(0.838633903678357,-0.0740444353928835,
0.508899795931835));
#15557=CARTESIAN_POINT('Ctrl Pts',(0.841298510752801,-0.0476299999999999,
0.504455939115715));
#15558=CARTESIAN_POINT('',(0.528110872004958,-0.04763,0.871530771444223));
#15559=CARTESIAN_POINT('Origin',(0.707106781186547,-0.04763,0.707106781186548));
#15560=CARTESIAN_POINT('',(0.871530771444223,-0.04763,0.528110872004959));
#15561=CARTESIAN_POINT('Ctrl Pts',(0.871530771444223,-0.0476300000000001,
0.528110872004958));
#15562=CARTESIAN_POINT('Ctrl Pts',(0.87014664509073,-0.0609922781173483,
0.530395067942936));
#15563=CARTESIAN_POINT('Ctrl Pts',(0.868149331745851,-0.0742967091364493,
0.533674141594226));
#15564=CARTESIAN_POINT('Ctrl Pts',(0.85981294420286,-0.115492077056649,
0.54708917182331));
#15565=CARTESIAN_POINT('Ctrl Pts',(0.850993704737257,-0.141695629206859,
0.560922177770136));
#15566=CARTESIAN_POINT('Ctrl Pts',(0.830754510485543,-0.181890537957859,
0.590422647829571));
#15567=CARTESIAN_POINT('Ctrl Pts',(0.816896541396381,-0.201072148666545,
0.609616703125488));
#15568=CARTESIAN_POINT('Ctrl Pts',(0.792310597819928,-0.223955109275652,
0.641117951819998));
#15569=CARTESIAN_POINT('Ctrl Pts',(0.779109323683612,-0.232742381310829,
0.657208095763053));
#15570=CARTESIAN_POINT('Ctrl Pts',(0.750552691816206,-0.244234834628584,
0.68964083160521));
#15571=CARTESIAN_POINT('Ctrl Pts',(0.735185187071673,-0.246942143572133,
0.705971972091755));
#15572=CARTESIAN_POINT('Ctrl Pts',(0.705971972091754,-0.246942143572133,
0.735185187071673));
#15573=CARTESIAN_POINT('Ctrl Pts',(0.689640831605209,-0.244234834628584,
0.750552691816206));
#15574=CARTESIAN_POINT('Ctrl Pts',(0.657208095763052,-0.232742381310829,
0.779109323683612));
#15575=CARTESIAN_POINT('Ctrl Pts',(0.641117951819998,-0.223955109275652,
0.792310597819928));
#15576=CARTESIAN_POINT('Ctrl Pts',(0.609616703125487,-0.201072148666545,
0.816896541396382));
#15577=CARTESIAN_POINT('Ctrl Pts',(0.590422647829571,-0.181890537957858,
0.830754510485544));
#15578=CARTESIAN_POINT('Ctrl Pts',(0.560922177770135,-0.141695629206858,
0.850993704737257));
#15579=CARTESIAN_POINT('Ctrl Pts',(0.547089171823309,-0.115492077056649,
0.859812944202861));
#15580=CARTESIAN_POINT('Ctrl Pts',(0.533674141594226,-0.0742967091364491,
0.868149331745852));
#15581=CARTESIAN_POINT('Ctrl Pts',(0.530395067942936,-0.0609922781173483,
0.870146645090731));
#15582=CARTESIAN_POINT('Ctrl Pts',(0.528110872004958,-0.0476300000000001,
0.871530771444223));
#15583=CARTESIAN_POINT('Origin',(0.707106781186547,-0.04763,0.707106781186548));
#15584=CARTESIAN_POINT('Origin',(0.,-0.166705,0.));
#15585=CARTESIAN_POINT('',(0.242834539687906,-0.04763,0.989696097314));
#15586=CARTESIAN_POINT('Origin',(0.,-0.04763,0.));
#15587=CARTESIAN_POINT('',(-0.242834539687907,-0.04763,0.989696097314));
#15588=CARTESIAN_POINT('Ctrl Pts',(0.242834539687906,-0.04763,0.989696097314));
#15589=CARTESIAN_POINT('Ctrl Pts',(0.24024064412003,-0.0609922781173483,
0.990332542620729));
#15590=CARTESIAN_POINT('Ctrl Pts',(0.236509675094874,-0.0742967091364492,
0.991238884025248));
#15591=CARTESIAN_POINT('Ctrl Pts',(0.221129100087819,-0.115492077056649,
0.994830026707808));
#15592=CARTESIAN_POINT('Ctrl Pts',(0.205111543747588,-0.141695629206859,
0.998375294985966));
#15593=CARTESIAN_POINT('Ctrl Pts',(0.169940289819232,-0.181890537957859,
1.00492400591205));
#15594=CARTESIAN_POINT('Ctrl Pts',(0.1465689792446,-0.201072148666545,1.00869718865384));
#15595=CARTESIAN_POINT('Ctrl Pts',(0.106909345252087,-0.223955109275652,
1.01358704779679));
#15596=CARTESIAN_POINT('Ctrl Pts',(0.0861971848975941,-0.232742381310829,
1.0156297872271));
#15597=CARTESIAN_POINT('Ctrl Pts',(0.0430711894098822,-0.244234834628584,
1.01837060663223));
#15598=CARTESIAN_POINT('Ctrl Pts',(0.0206568624125605,-0.246942143572133,
1.019052));
#15599=CARTESIAN_POINT('Ctrl Pts',(-0.0206568624125608,-0.246942143572133,
1.019052));
#15600=CARTESIAN_POINT('Ctrl Pts',(-0.0430711894098825,-0.244234834628584,
1.01837060663223));
#15601=CARTESIAN_POINT('Ctrl Pts',(-0.0861971848975943,-0.232742381310829,
1.0156297872271));
#15602=CARTESIAN_POINT('Ctrl Pts',(-0.106909345252088,-0.223955109275652,
1.01358704779679));
#15603=CARTESIAN_POINT('Ctrl Pts',(-0.1465689792446,-0.201072148666545,
1.00869718865384));
#15604=CARTESIAN_POINT('Ctrl Pts',(-0.169940289819232,-0.181890537957859,
1.00492400591205));
#15605=CARTESIAN_POINT('Ctrl Pts',(-0.205111543747588,-0.141695629206859,
0.998375294985966));
#15606=CARTESIAN_POINT('Ctrl Pts',(-0.221129100087819,-0.115492077056649,
0.994830026707808));
#15607=CARTESIAN_POINT('Ctrl Pts',(-0.236509675094875,-0.0742967091364493,
0.991238884025248));
#15608=CARTESIAN_POINT('Ctrl Pts',(-0.24024064412003,-0.0609922781173483,
0.990332542620729));
#15609=CARTESIAN_POINT('Ctrl Pts',(-0.242834539687907,-0.04763,0.989696097314));
#15610=CARTESIAN_POINT('',(-0.528110872004959,-0.04763,0.871530771444223));
#15611=CARTESIAN_POINT('Origin',(0.,-0.04763,0.));
#15612=CARTESIAN_POINT('',(-0.871530771444223,-0.04763,0.528110872004958));
#15613=CARTESIAN_POINT('Ctrl Pts',(-0.528110872004958,-0.0476300000000001,
0.871530771444223));
#15614=CARTESIAN_POINT('Ctrl Pts',(-0.530395067942936,-0.0609922781173484,
0.87014664509073));
#15615=CARTESIAN_POINT('Ctrl Pts',(-0.533674141594226,-0.0742967091364493,
0.868149331745851));
#15616=CARTESIAN_POINT('Ctrl Pts',(-0.54708917182331,-0.115492077056649,
0.85981294420286));
#15617=CARTESIAN_POINT('Ctrl Pts',(-0.560922177770136,-0.141695629206859,
0.850993704737257));
#15618=CARTESIAN_POINT('Ctrl Pts',(-0.590422647829571,-0.181890537957859,
0.830754510485543));
#15619=CARTESIAN_POINT('Ctrl Pts',(-0.609616703125488,-0.201072148666545,
0.816896541396381));
#15620=CARTESIAN_POINT('Ctrl Pts',(-0.641117951819998,-0.223955109275652,
0.792310597819928));
#15621=CARTESIAN_POINT('Ctrl Pts',(-0.657208095763053,-0.232742381310829,
0.779109323683611));
#15622=CARTESIAN_POINT('Ctrl Pts',(-0.68964083160521,-0.244234834628584,
0.750552691816205));
#15623=CARTESIAN_POINT('Ctrl Pts',(-0.705971972091755,-0.246942143572133,
0.735185187071673));
#15624=CARTESIAN_POINT('Ctrl Pts',(-0.735185187071673,-0.246942143572133,
0.705971972091754));
#15625=CARTESIAN_POINT('Ctrl Pts',(-0.750552691816206,-0.244234834628584,
0.689640831605209));
#15626=CARTESIAN_POINT('Ctrl Pts',(-0.779109323683612,-0.232742381310829,
0.657208095763052));
#15627=CARTESIAN_POINT('Ctrl Pts',(-0.792310597819928,-0.223955109275652,
0.641117951819998));
#15628=CARTESIAN_POINT('Ctrl Pts',(-0.816896541396382,-0.201072148666545,
0.609616703125487));
#15629=CARTESIAN_POINT('Ctrl Pts',(-0.830754510485544,-0.181890537957858,
0.590422647829571));
#15630=CARTESIAN_POINT('Ctrl Pts',(-0.850993704737257,-0.141695629206858,
0.560922177770135));
#15631=CARTESIAN_POINT('Ctrl Pts',(-0.859812944202861,-0.115492077056649,
0.547089171823309));
#15632=CARTESIAN_POINT('Ctrl Pts',(-0.868149331745852,-0.0742967091364491,
0.533674141594226));
#15633=CARTESIAN_POINT('Ctrl Pts',(-0.870146645090731,-0.0609922781173483,
0.530395067942936));
#15634=CARTESIAN_POINT('Ctrl Pts',(-0.871530771444223,-0.04763,0.528110872004958));
#15635=CARTESIAN_POINT('',(-0.989696097314,-0.04763,0.242834539687906));
#15636=CARTESIAN_POINT('Origin',(0.,-0.04763,0.));
#15637=CARTESIAN_POINT('',(-1.019052,-0.246942143572133,1.248489836334E-16));
#15638=CARTESIAN_POINT('Ctrl Pts',(-0.989696097314,-0.04763,0.242834539687906));
#15639=CARTESIAN_POINT('Ctrl Pts',(-0.990332542620729,-0.0609922781173483,
0.24024064412003));
#15640=CARTESIAN_POINT('Ctrl Pts',(-0.991238884025248,-0.0742967091364492,
0.236509675094874));
#15641=CARTESIAN_POINT('Ctrl Pts',(-0.994830026707808,-0.115492077056649,
0.221129100087819));
#15642=CARTESIAN_POINT('Ctrl Pts',(-0.998375294985966,-0.141695629206859,
0.205111543747588));
#15643=CARTESIAN_POINT('Ctrl Pts',(-1.00492400591205,-0.181890537957859,
0.169940289819232));
#15644=CARTESIAN_POINT('Ctrl Pts',(-1.00869718865384,-0.201072148666545,
0.1465689792446));
#15645=CARTESIAN_POINT('Ctrl Pts',(-1.01358704779679,-0.223955109275652,
0.106909345252088));
#15646=CARTESIAN_POINT('Ctrl Pts',(-1.0156297872271,-0.232742381310829,
0.0861971848975944));
#15647=CARTESIAN_POINT('Ctrl Pts',(-1.01837060663223,-0.244234834628584,
0.0430711894098825));
#15648=CARTESIAN_POINT('Ctrl Pts',(-1.019052,-0.246942143572133,0.0206568624125608));
#15649=CARTESIAN_POINT('Ctrl Pts',(-1.019052,-0.246942143572133,1.2490009027033E-16));
#15650=CARTESIAN_POINT('',(-1.019052,-0.28578,1.24797876996471E-16));
#15651=CARTESIAN_POINT('',(-1.019052,-0.166705,1.24797876996471E-16));
#15652=CARTESIAN_POINT('Origin',(0.,-0.28578,0.));
#15653=CARTESIAN_POINT('',(-0.989696097314,-0.04763,-0.242834539687906));
#15654=CARTESIAN_POINT('Ctrl Pts',(-1.019052,-0.246942143572133,1.2490009027033E-16));
#15655=CARTESIAN_POINT('Ctrl Pts',(-1.019052,-0.246942143572133,-0.0206568624125605));
#15656=CARTESIAN_POINT('Ctrl Pts',(-1.01837060663223,-0.244234834628584,
-0.0430711894098822));
#15657=CARTESIAN_POINT('Ctrl Pts',(-1.0156297872271,-0.232742381310829,
-0.0861971848975941));
#15658=CARTESIAN_POINT('Ctrl Pts',(-1.01358704779679,-0.223955109275652,
-0.106909345252087));
#15659=CARTESIAN_POINT('Ctrl Pts',(-1.00869718865384,-0.201072148666546,
-0.1465689792446));
#15660=CARTESIAN_POINT('Ctrl Pts',(-1.00492400591205,-0.181890537957859,
-0.169940289819232));
#15661=CARTESIAN_POINT('Ctrl Pts',(-0.998375294985966,-0.141695629206859,
-0.205111543747588));
#15662=CARTESIAN_POINT('Ctrl Pts',(-0.994830026707808,-0.11549207705665,
-0.221129100087819));
#15663=CARTESIAN_POINT('Ctrl Pts',(-0.991238884025248,-0.0742967091364495,
-0.236509675094874));
#15664=CARTESIAN_POINT('Ctrl Pts',(-0.990332542620729,-0.0609922781173484,
-0.24024064412003));
#15665=CARTESIAN_POINT('Ctrl Pts',(-0.989696097314,-0.0476300000000001,
-0.242834539687907));
#15666=CARTESIAN_POINT('',(-0.871530771444223,-0.04763,-0.528110872004958));
#15667=CARTESIAN_POINT('Origin',(0.,-0.04763,0.));
#15668=CARTESIAN_POINT('',(-0.528110872004958,-0.04763,-0.871530771444223));
#15669=CARTESIAN_POINT('Ctrl Pts',(-0.871530771444223,-0.0476300000000001,
-0.528110872004958));
#15670=CARTESIAN_POINT('Ctrl Pts',(-0.87014664509073,-0.0609922781173484,
-0.530395067942936));
#15671=CARTESIAN_POINT('Ctrl Pts',(-0.868149331745851,-0.0742967091364494,
-0.533674141594226));
#15672=CARTESIAN_POINT('Ctrl Pts',(-0.85981294420286,-0.115492077056649,
-0.54708917182331));
#15673=CARTESIAN_POINT('Ctrl Pts',(-0.850993704737257,-0.141695629206859,
-0.560922177770136));
#15674=CARTESIAN_POINT('Ctrl Pts',(-0.830754510485543,-0.181890537957859,
-0.590422647829571));
#15675=CARTESIAN_POINT('Ctrl Pts',(-0.816896541396381,-0.201072148666546,
-0.609616703125488));
#15676=CARTESIAN_POINT('Ctrl Pts',(-0.792310597819928,-0.223955109275652,
-0.641117951819999));
#15677=CARTESIAN_POINT('Ctrl Pts',(-0.779109323683611,-0.232742381310829,
-0.657208095763053));
#15678=CARTESIAN_POINT('Ctrl Pts',(-0.750552691816205,-0.244234834628584,
-0.68964083160521));
#15679=CARTESIAN_POINT('Ctrl Pts',(-0.735185187071673,-0.246942143572133,
-0.705971972091755));
#15680=CARTESIAN_POINT('Ctrl Pts',(-0.705971972091754,-0.246942143572133,
-0.735185187071673));
#15681=CARTESIAN_POINT('Ctrl Pts',(-0.68964083160521,-0.244234834628584,
-0.750552691816206));
#15682=CARTESIAN_POINT('Ctrl Pts',(-0.657208095763052,-0.232742381310829,
-0.779109323683612));
#15683=CARTESIAN_POINT('Ctrl Pts',(-0.641117951819998,-0.223955109275652,
-0.792310597819928));
#15684=CARTESIAN_POINT('Ctrl Pts',(-0.609616703125488,-0.201072148666545,
-0.816896541396381));
#15685=CARTESIAN_POINT('Ctrl Pts',(-0.590422647829571,-0.181890537957859,
-0.830754510485543));
#15686=CARTESIAN_POINT('Ctrl Pts',(-0.560922177770136,-0.141695629206859,
-0.850993704737257));
#15687=CARTESIAN_POINT('Ctrl Pts',(-0.54708917182331,-0.115492077056649,
-0.85981294420286));
#15688=CARTESIAN_POINT('Ctrl Pts',(-0.533674141594226,-0.0742967091364494,
-0.868149331745852));
#15689=CARTESIAN_POINT('Ctrl Pts',(-0.530395067942936,-0.0609922781173484,
-0.870146645090731));
#15690=CARTESIAN_POINT('Ctrl Pts',(-0.528110872004958,-0.0476300000000001,
-0.871530771444223));
#15691=CARTESIAN_POINT('',(-0.242834539687906,-0.04763,-0.989696097314));
#15692=CARTESIAN_POINT('Origin',(0.,-0.04763,0.));
#15693=CARTESIAN_POINT('',(0.242834539687906,-0.04763,-0.989696097314));
#15694=CARTESIAN_POINT('Ctrl Pts',(-0.242834539687907,-0.04763,-0.989696097314));
#15695=CARTESIAN_POINT('Ctrl Pts',(-0.24024064412003,-0.0609922781173483,
-0.990332542620729));
#15696=CARTESIAN_POINT('Ctrl Pts',(-0.236509675094874,-0.0742967091364493,
-0.991238884025248));
#15697=CARTESIAN_POINT('Ctrl Pts',(-0.221129100087819,-0.115492077056649,
-0.994830026707808));
#15698=CARTESIAN_POINT('Ctrl Pts',(-0.205111543747588,-0.141695629206859,
-0.998375294985966));
#15699=CARTESIAN_POINT('Ctrl Pts',(-0.169940289819232,-0.181890537957859,
-1.00492400591205));
#15700=CARTESIAN_POINT('Ctrl Pts',(-0.1465689792446,-0.201072148666545,
-1.00869718865384));
#15701=CARTESIAN_POINT('Ctrl Pts',(-0.106909345252087,-0.223955109275652,
-1.01358704779679));
#15702=CARTESIAN_POINT('Ctrl Pts',(-0.0861971848975942,-0.232742381310829,
-1.0156297872271));
#15703=CARTESIAN_POINT('Ctrl Pts',(-0.0430711894098823,-0.244234834628584,
-1.01837060663223));
#15704=CARTESIAN_POINT('Ctrl Pts',(-0.0206568624125606,-0.246942143572133,
-1.019052));
#15705=CARTESIAN_POINT('Ctrl Pts',(0.0206568624125607,-0.246942143572133,
-1.019052));
#15706=CARTESIAN_POINT('Ctrl Pts',(0.0430711894098824,-0.244234834628584,
-1.01837060663223));
#15707=CARTESIAN_POINT('Ctrl Pts',(0.0861971848975943,-0.232742381310829,
-1.0156297872271));
#15708=CARTESIAN_POINT('Ctrl Pts',(0.106909345252088,-0.223955109275652,
-1.01358704779679));
#15709=CARTESIAN_POINT('Ctrl Pts',(0.1465689792446,-0.201072148666545,-1.00869718865384));
#15710=CARTESIAN_POINT('Ctrl Pts',(0.169940289819232,-0.181890537957859,
-1.00492400591205));
#15711=CARTESIAN_POINT('Ctrl Pts',(0.205111543747588,-0.141695629206859,
-0.998375294985966));
#15712=CARTESIAN_POINT('Ctrl Pts',(0.221129100087819,-0.115492077056649,
-0.994830026707808));
#15713=CARTESIAN_POINT('Ctrl Pts',(0.236509675094874,-0.0742967091364493,
-0.991238884025248));
#15714=CARTESIAN_POINT('Ctrl Pts',(0.24024064412003,-0.0609922781173484,
-0.990332542620729));
#15715=CARTESIAN_POINT('Ctrl Pts',(0.242834539687907,-0.04763,-0.989696097314));
#15716=CARTESIAN_POINT('',(0.528110872004958,-0.04763,-0.871530771444223));
#15717=CARTESIAN_POINT('Origin',(0.,-0.04763,0.));
#15718=CARTESIAN_POINT('',(0.871530771444223,-0.04763,-0.528110872004958));
#15719=CARTESIAN_POINT('Ctrl Pts',(0.528110872004958,-0.0476300000000001,
-0.871530771444223));
#15720=CARTESIAN_POINT('Ctrl Pts',(0.530395067942936,-0.0609922781173484,
-0.870146645090731));
#15721=CARTESIAN_POINT('Ctrl Pts',(0.533674141594226,-0.0742967091364493,
-0.868149331745851));
#15722=CARTESIAN_POINT('Ctrl Pts',(0.54708917182331,-0.115492077056649,
-0.85981294420286));
#15723=CARTESIAN_POINT('Ctrl Pts',(0.560922177770136,-0.141695629206859,
-0.850993704737257));
#15724=CARTESIAN_POINT('Ctrl Pts',(0.590422647829571,-0.181890537957859,
-0.830754510485543));
#15725=CARTESIAN_POINT('Ctrl Pts',(0.609616703125488,-0.201072148666545,
-0.816896541396381));
#15726=CARTESIAN_POINT('Ctrl Pts',(0.641117951819998,-0.223955109275652,
-0.792310597819928));
#15727=CARTESIAN_POINT('Ctrl Pts',(0.657208095763053,-0.232742381310829,
-0.779109323683612));
#15728=CARTESIAN_POINT('Ctrl Pts',(0.68964083160521,-0.244234834628584,
-0.750552691816206));
#15729=CARTESIAN_POINT('Ctrl Pts',(0.705971972091755,-0.246942143572133,
-0.735185187071673));
#15730=CARTESIAN_POINT('Ctrl Pts',(0.735185187071673,-0.246942143572133,
-0.705971972091754));
#15731=CARTESIAN_POINT('Ctrl Pts',(0.750552691816206,-0.244234834628584,
-0.68964083160521));
#15732=CARTESIAN_POINT('Ctrl Pts',(0.779109323683612,-0.232742381310829,
-0.657208095763053));
#15733=CARTESIAN_POINT('Ctrl Pts',(0.792310597819928,-0.223955109275652,
-0.641117951819998));
#15734=CARTESIAN_POINT('Ctrl Pts',(0.816896541396381,-0.201072148666545,
-0.609616703125488));
#15735=CARTESIAN_POINT('Ctrl Pts',(0.830754510485543,-0.181890537957859,
-0.590422647829571));
#15736=CARTESIAN_POINT('Ctrl Pts',(0.850993704737257,-0.141695629206859,
-0.560922177770136));
#15737=CARTESIAN_POINT('Ctrl Pts',(0.85981294420286,-0.115492077056649,
-0.54708917182331));
#15738=CARTESIAN_POINT('Ctrl Pts',(0.868149331745851,-0.0742967091364493,
-0.533674141594226));
#15739=CARTESIAN_POINT('Ctrl Pts',(0.870146645090731,-0.0609922781173484,
-0.530395067942936));
#15740=CARTESIAN_POINT('Ctrl Pts',(0.871530771444223,-0.0476300000000001,
-0.528110872004958));
#15741=CARTESIAN_POINT('',(0.989696097314,-0.04763,-0.242834539687906));
#15742=CARTESIAN_POINT('Origin',(0.,-0.04763,0.));
#15743=CARTESIAN_POINT('',(0.989696097314,-0.04763,0.242834539687906));
#15744=CARTESIAN_POINT('Ctrl Pts',(0.989696097314,-0.04763,-0.242834539687907));
#15745=CARTESIAN_POINT('Ctrl Pts',(0.990332542620729,-0.0609922781173483,
-0.24024064412003));
#15746=CARTESIAN_POINT('Ctrl Pts',(0.991238884025248,-0.0742967091364493,
-0.236509675094874));
#15747=CARTESIAN_POINT('Ctrl Pts',(0.994830026707808,-0.115492077056649,
-0.221129100087819));
#15748=CARTESIAN_POINT('Ctrl Pts',(0.998375294985966,-0.141695629206859,
-0.205111543747588));
#15749=CARTESIAN_POINT('Ctrl Pts',(1.00492400591205,-0.181890537957859,
-0.169940289819232));
#15750=CARTESIAN_POINT('Ctrl Pts',(1.00869718865384,-0.201072148666545,
-0.1465689792446));
#15751=CARTESIAN_POINT('Ctrl Pts',(1.01358704779679,-0.223955109275652,
-0.106909345252087));
#15752=CARTESIAN_POINT('Ctrl Pts',(1.0156297872271,-0.232742381310829,-0.0861971848975942));
#15753=CARTESIAN_POINT('Ctrl Pts',(1.01837060663223,-0.244234834628584,
-0.0430711894098823));
#15754=CARTESIAN_POINT('Ctrl Pts',(1.019052,-0.246942143572133,-0.0206568624125607));
#15755=CARTESIAN_POINT('Ctrl Pts',(1.019052,-0.246942143572133,0.0206568624125607));
#15756=CARTESIAN_POINT('Ctrl Pts',(1.01837060663223,-0.244234834628584,
0.0430711894098823));
#15757=CARTESIAN_POINT('Ctrl Pts',(1.0156297872271,-0.232742381310829,0.0861971848975942));
#15758=CARTESIAN_POINT('Ctrl Pts',(1.01358704779679,-0.223955109275652,
0.106909345252087));
#15759=CARTESIAN_POINT('Ctrl Pts',(1.00869718865384,-0.201072148666545,
0.1465689792446));
#15760=CARTESIAN_POINT('Ctrl Pts',(1.00492400591205,-0.181890537957859,
0.169940289819232));
#15761=CARTESIAN_POINT('Ctrl Pts',(0.998375294985966,-0.141695629206859,
0.205111543747588));
#15762=CARTESIAN_POINT('Ctrl Pts',(0.994830026707808,-0.115492077056649,
0.221129100087819));
#15763=CARTESIAN_POINT('Ctrl Pts',(0.991238884025248,-0.0742967091364492,
0.236509675094874));
#15764=CARTESIAN_POINT('Ctrl Pts',(0.990332542620729,-0.0609922781173483,
0.24024064412003));
#15765=CARTESIAN_POINT('Ctrl Pts',(0.989696097314,-0.04763,0.242834539687907));
#15766=CARTESIAN_POINT('Origin',(0.,-0.04763,0.));
#15767=CARTESIAN_POINT('Origin',(0.,-0.04763,0.));
#15768=CARTESIAN_POINT('',(0.238183666596899,-0.04763,0.951592097314));
#15769=CARTESIAN_POINT('Origin',(0.,-0.04763,0.));
#15770=CARTESIAN_POINT('Origin',(-1.94289029309402E-16,-0.04763,1.));
#15771=CARTESIAN_POINT('Origin',(-1.94289029309402E-16,0.,1.));
#15772=CARTESIAN_POINT('',(-0.2381836665969,-0.04763,0.951592097314));
#15773=CARTESIAN_POINT('Ctrl Pts',(-0.238183666596899,-0.0476299999999999,
0.951592097314));
#15774=CARTESIAN_POINT('Ctrl Pts',(-0.233157223576062,-0.0740444353928835,
0.952850216871763));
#15775=CARTESIAN_POINT('Ctrl Pts',(-0.223801617934946,-0.0999305678883309,
0.955173119738174));
#15776=CARTESIAN_POINT('Ctrl Pts',(-0.199966927975188,-0.142345102874864,
0.960411259488514));
#15777=CARTESIAN_POINT('Ctrl Pts',(-0.1868781821531,-0.159766064500479,
0.963103647174702));
#15778=CARTESIAN_POINT('Ctrl Pts',(-0.15681442133453,-0.190326085855194,
0.968453058988463));
#15779=CARTESIAN_POINT('Ctrl Pts',(-0.139836317888043,-0.203463743702801,
0.971100730005489));
#15780=CARTESIAN_POINT('Ctrl Pts',(-0.104422493053067,-0.224161999508995,
0.975530745318961));
#15781=CARTESIAN_POINT('Ctrl Pts',(-0.0842175114474176,-0.232861760990032,
0.977553872336861));
#15782=CARTESIAN_POINT('Ctrl Pts',(-0.0421062857595701,-0.244251601209411,
0.980270995488453));
#15783=CARTESIAN_POINT('Ctrl Pts',(-0.0201990724523197,-0.246942143572133,
0.980948));
#15784=CARTESIAN_POINT('Ctrl Pts',(0.020199072452319,-0.246942143572133,
0.980948));
#15785=CARTESIAN_POINT('Ctrl Pts',(0.0421062857595694,-0.244251601209411,
0.980270995488454));
#15786=CARTESIAN_POINT('Ctrl Pts',(0.0842175114474169,-0.232861760990032,
0.977553872336861));
#15787=CARTESIAN_POINT('Ctrl Pts',(0.104422493053067,-0.224161999508995,
0.975530745318961));
#15788=CARTESIAN_POINT('Ctrl Pts',(0.139836317888042,-0.203463743702801,
0.971100730005489));
#15789=CARTESIAN_POINT('Ctrl Pts',(0.15681442133453,-0.190326085855194,
0.968453058988463));
#15790=CARTESIAN_POINT('Ctrl Pts',(0.1868781821531,-0.15976606450048,0.963103647174702));
#15791=CARTESIAN_POINT('Ctrl Pts',(0.199966927975188,-0.142345102874864,
0.960411259488514));
#15792=CARTESIAN_POINT('Ctrl Pts',(0.223801617934945,-0.0999305678883309,
0.955173119738174));
#15793=CARTESIAN_POINT('Ctrl Pts',(0.233157223576061,-0.0740444353928835,
0.952850216871763));
#15794=CARTESIAN_POINT('Ctrl Pts',(0.238183666596899,-0.0476299999999999,
0.951592097314));
#15795=CARTESIAN_POINT('Origin',(-1.94289029309402E-16,-0.04763,1.));
#15796=CARTESIAN_POINT('Origin',(0.,-0.04763,0.));
#15797=CARTESIAN_POINT('',(-0.504455939115715,-0.04763,0.841298510752802));
#15798=CARTESIAN_POINT('Origin',(0.,-0.04763,0.));
#15799=CARTESIAN_POINT('Origin',(-0.707106781186548,-0.04763,0.707106781186547));
#15800=CARTESIAN_POINT('Origin',(-0.707106781186548,0.,0.707106781186547));
#15801=CARTESIAN_POINT('',(-0.841298510752802,-0.04763,0.504455939115715));
#15802=CARTESIAN_POINT('Ctrl Pts',(-0.841298510752802,-0.04763,0.504455939115715));
#15803=CARTESIAN_POINT('Ctrl Pts',(-0.838633903678357,-0.0740444353928835,
0.508899795931835));
#15804=CARTESIAN_POINT('Ctrl Pts',(-0.833661031856294,-0.0999305678883309,
0.517157748491652));
#15805=CARTESIAN_POINT('Ctrl Pts',(-0.820511285096538,-0.142345102874864,
0.537715343527944));
#15806=CARTESIAN_POINT('Ctrl Pts',(-0.813159949759,-0.159766064500479,0.548874290046456));
#15807=CARTESIAN_POINT('Ctrl Pts',(-0.795684265985089,-0.190326085855194,
0.573915184558107));
#15808=CARTESIAN_POINT('Ctrl Pts',(-0.78555112003688,-0.203463743702801,
0.587792702767295));
#15809=CARTESIAN_POINT('Ctrl Pts',(-0.763642258217233,-0.224161999508995,
0.615966552324775));
#15810=CARTESIAN_POINT('Ctrl Pts',(-0.750785745543687,-0.232861760990032,
0.631684198665438));
#15811=CARTESIAN_POINT('Ctrl Pts',(-0.722929908501543,-0.244251601209411,
0.663382628119203));
#15812=CARTESIAN_POINT('Ctrl Pts',(-0.707917883896095,-0.246942143572133,
0.679352081686668));
#15813=CARTESIAN_POINT('Ctrl Pts',(-0.679352081686668,-0.246942143572133,
0.707917883896095));
#15814=CARTESIAN_POINT('Ctrl Pts',(-0.663382628119203,-0.244251601209411,
0.722929908501544));
#15815=CARTESIAN_POINT('Ctrl Pts',(-0.631684198665438,-0.232861760990031,
0.750785745543687));
#15816=CARTESIAN_POINT('Ctrl Pts',(-0.615966552324775,-0.224161999508995,
0.763642258217233));
#15817=CARTESIAN_POINT('Ctrl Pts',(-0.587792702767295,-0.203463743702801,
0.78555112003688));
#15818=CARTESIAN_POINT('Ctrl Pts',(-0.573915184558107,-0.190326085855194,
0.795684265985088));
#15819=CARTESIAN_POINT('Ctrl Pts',(-0.548874290046456,-0.159766064500479,
0.813159949759));
#15820=CARTESIAN_POINT('Ctrl Pts',(-0.537715343527944,-0.142345102874864,
0.820511285096538));
#15821=CARTESIAN_POINT('Ctrl Pts',(-0.517157748491652,-0.0999305678883309,
0.833661031856294));
#15822=CARTESIAN_POINT('Ctrl Pts',(-0.508899795931835,-0.0740444353928835,
0.838633903678357));
#15823=CARTESIAN_POINT('Ctrl Pts',(-0.504455939115716,-0.04763,0.841298510752801));
#15824=CARTESIAN_POINT('Origin',(-0.707106781186548,-0.04763,0.707106781186547));
#15825=CARTESIAN_POINT('Origin',(0.,-0.04763,0.));
#15826=CARTESIAN_POINT('',(-0.951592097314,-0.04763,0.238183666596899));
#15827=CARTESIAN_POINT('Origin',(0.,-0.04763,0.));
#15828=CARTESIAN_POINT('Origin',(-1.,-0.04763,-1.11022302462516E-16));
#15829=CARTESIAN_POINT('Origin',(-1.,0.,-1.11022302462516E-16));
#15830=CARTESIAN_POINT('',(-0.951592097314,-0.04763,-0.2381836665969));
#15831=CARTESIAN_POINT('',(-0.980948,-0.246942143572133,1.08514323328844E-18));
#15832=CARTESIAN_POINT('Ctrl Pts',(-0.951592097314,-0.04763,-0.238183666596899));
#15833=CARTESIAN_POINT('Ctrl Pts',(-0.952850216871763,-0.0740444353928835,
-0.233157223576062));
#15834=CARTESIAN_POINT('Ctrl Pts',(-0.955173119738174,-0.0999305678883309,
-0.223801617934946));
#15835=CARTESIAN_POINT('Ctrl Pts',(-0.960411259488514,-0.142345102874864,
-0.199966927975188));
#15836=CARTESIAN_POINT('Ctrl Pts',(-0.963103647174702,-0.159766064500479,
-0.1868781821531));
#15837=CARTESIAN_POINT('Ctrl Pts',(-0.968453058988463,-0.190326085855194,
-0.15681442133453));
#15838=CARTESIAN_POINT('Ctrl Pts',(-0.971100730005489,-0.203463743702801,
-0.139836317888043));
#15839=CARTESIAN_POINT('Ctrl Pts',(-0.975530745318961,-0.224161999508995,
-0.104422493053067));
#15840=CARTESIAN_POINT('Ctrl Pts',(-0.977553872336861,-0.232861760990032,
-0.0842175114474175));
#15841=CARTESIAN_POINT('Ctrl Pts',(-0.980270995488453,-0.244251601209411,
-0.0421062857595699));
#15842=CARTESIAN_POINT('Ctrl Pts',(-0.980948,-0.246942143572133,-0.0201990724523195));
#15843=CARTESIAN_POINT('Ctrl Pts',(-0.980948,-0.246942143572133,-1.17961196366423E-16));
#15844=CARTESIAN_POINT('Origin',(-1.,-0.04763,-1.11022302462516E-16));
#15845=CARTESIAN_POINT('Ctrl Pts',(-0.980948,-0.246942143572133,-1.17961196366423E-16));
#15846=CARTESIAN_POINT('Ctrl Pts',(-0.980948,-0.246942143572133,0.0201990724523192));
#15847=CARTESIAN_POINT('Ctrl Pts',(-0.980270995488453,-0.244251601209411,
0.0421062857595695));
#15848=CARTESIAN_POINT('Ctrl Pts',(-0.977553872336861,-0.232861760990032,
0.0842175114474169));
#15849=CARTESIAN_POINT('Ctrl Pts',(-0.975530745318961,-0.224161999508995,
0.104422493053066));
#15850=CARTESIAN_POINT('Ctrl Pts',(-0.971100730005489,-0.203463743702801,
0.139836317888042));
#15851=CARTESIAN_POINT('Ctrl Pts',(-0.968453058988463,-0.190326085855194,
0.15681442133453));
#15852=CARTESIAN_POINT('Ctrl Pts',(-0.963103647174702,-0.15976606450048,
0.1868781821531));
#15853=CARTESIAN_POINT('Ctrl Pts',(-0.960411259488514,-0.142345102874864,
0.199966927975188));
#15854=CARTESIAN_POINT('Ctrl Pts',(-0.955173119738174,-0.099930567888331,
0.223801617934945));
#15855=CARTESIAN_POINT('Ctrl Pts',(-0.952850216871763,-0.0740444353928835,
0.233157223576061));
#15856=CARTESIAN_POINT('Ctrl Pts',(-0.951592097314,-0.04763,0.238183666596899));
#15857=CARTESIAN_POINT('Origin',(0.,-0.04763,0.));
#15858=CARTESIAN_POINT('',(-0.841298510752802,-0.04763,-0.504455939115715));
#15859=CARTESIAN_POINT('Origin',(0.,-0.04763,0.));
#15860=CARTESIAN_POINT('Origin',(-0.707106781186547,-0.04763,-0.707106781186548));
#15861=CARTESIAN_POINT('Origin',(-0.707106781186547,0.,-0.707106781186548));
#15862=CARTESIAN_POINT('',(-0.504455939115715,-0.04763,-0.841298510752802));
#15863=CARTESIAN_POINT('Ctrl Pts',(-0.504455939115715,-0.04763,-0.841298510752802));
#15864=CARTESIAN_POINT('Ctrl Pts',(-0.508899795931835,-0.0740444353928835,
-0.838633903678357));
#15865=CARTESIAN_POINT('Ctrl Pts',(-0.517157748491652,-0.0999305678883309,
-0.833661031856294));
#15866=CARTESIAN_POINT('Ctrl Pts',(-0.537715343527944,-0.142345102874864,
-0.820511285096538));
#15867=CARTESIAN_POINT('Ctrl Pts',(-0.548874290046456,-0.159766064500479,
-0.813159949759));
#15868=CARTESIAN_POINT('Ctrl Pts',(-0.573915184558107,-0.190326085855194,
-0.795684265985089));
#15869=CARTESIAN_POINT('Ctrl Pts',(-0.587792702767295,-0.203463743702801,
-0.78555112003688));
#15870=CARTESIAN_POINT('Ctrl Pts',(-0.615966552324775,-0.224161999508995,
-0.763642258217233));
#15871=CARTESIAN_POINT('Ctrl Pts',(-0.631684198665438,-0.232861760990032,
-0.750785745543687));
#15872=CARTESIAN_POINT('Ctrl Pts',(-0.663382628119203,-0.244251601209411,
-0.722929908501543));
#15873=CARTESIAN_POINT('Ctrl Pts',(-0.679352081686668,-0.246942143572133,
-0.707917883896095));
#15874=CARTESIAN_POINT('Ctrl Pts',(-0.707917883896095,-0.246942143572133,
-0.679352081686668));
#15875=CARTESIAN_POINT('Ctrl Pts',(-0.722929908501543,-0.244251601209411,
-0.663382628119203));
#15876=CARTESIAN_POINT('Ctrl Pts',(-0.750785745543687,-0.232861760990032,
-0.631684198665439));
#15877=CARTESIAN_POINT('Ctrl Pts',(-0.763642258217232,-0.224161999508995,
-0.615966552324775));
#15878=CARTESIAN_POINT('Ctrl Pts',(-0.78555112003688,-0.203463743702801,
-0.587792702767295));
#15879=CARTESIAN_POINT('Ctrl Pts',(-0.795684265985088,-0.190326085855194,
-0.573915184558107));
#15880=CARTESIAN_POINT('Ctrl Pts',(-0.813159949759,-0.15976606450048,-0.548874290046456));
#15881=CARTESIAN_POINT('Ctrl Pts',(-0.820511285096538,-0.142345102874864,
-0.537715343527944));
#15882=CARTESIAN_POINT('Ctrl Pts',(-0.833661031856294,-0.0999305678883311,
-0.517157748491652));
#15883=CARTESIAN_POINT('Ctrl Pts',(-0.838633903678357,-0.0740444353928836,
-0.508899795931835));
#15884=CARTESIAN_POINT('Ctrl Pts',(-0.841298510752801,-0.04763,-0.504455939115715));
#15885=CARTESIAN_POINT('Origin',(-0.707106781186547,-0.04763,-0.707106781186548));
#15886=CARTESIAN_POINT('Origin',(0.,-0.04763,0.));
#15887=CARTESIAN_POINT('',(-0.238183666596899,-0.04763,-0.951592097314));
#15888=CARTESIAN_POINT('Origin',(0.,-0.04763,0.));
#15889=CARTESIAN_POINT('Origin',(5.55111512312578E-17,-0.04763,-1.));
#15890=CARTESIAN_POINT('Origin',(5.55111512312578E-17,0.,-1.));
#15891=CARTESIAN_POINT('',(0.238183666596899,-0.04763,-0.951592097314));
#15892=CARTESIAN_POINT('Ctrl Pts',(0.238183666596899,-0.04763,-0.951592097314));
#15893=CARTESIAN_POINT('Ctrl Pts',(0.233157223576062,-0.0740444353928835,
-0.952850216871763));
#15894=CARTESIAN_POINT('Ctrl Pts',(0.223801617934946,-0.099930567888331,
-0.955173119738174));
#15895=CARTESIAN_POINT('Ctrl Pts',(0.199966927975188,-0.142345102874864,
-0.960411259488514));
#15896=CARTESIAN_POINT('Ctrl Pts',(0.1868781821531,-0.15976606450048,-0.963103647174702));
#15897=CARTESIAN_POINT('Ctrl Pts',(0.15681442133453,-0.190326085855194,
-0.968453058988463));
#15898=CARTESIAN_POINT('Ctrl Pts',(0.139836317888042,-0.203463743702801,
-0.971100730005489));
#15899=CARTESIAN_POINT('Ctrl Pts',(0.104422493053067,-0.224161999508995,
-0.975530745318961));
#15900=CARTESIAN_POINT('Ctrl Pts',(0.0842175114474173,-0.232861760990032,
-0.977553872336861));
#15901=CARTESIAN_POINT('Ctrl Pts',(0.0421062857595698,-0.244251601209411,
-0.980270995488453));
#15902=CARTESIAN_POINT('Ctrl Pts',(0.0201990724523194,-0.246942143572133,
-0.980948));
#15903=CARTESIAN_POINT('Ctrl Pts',(-0.0201990724523193,-0.246942143572133,
-0.980948));
#15904=CARTESIAN_POINT('Ctrl Pts',(-0.0421062857595697,-0.244251601209411,
-0.980270995488453));
#15905=CARTESIAN_POINT('Ctrl Pts',(-0.0842175114474171,-0.232861760990032,
-0.977553872336861));
#15906=CARTESIAN_POINT('Ctrl Pts',(-0.104422493053067,-0.224161999508995,
-0.975530745318961));
#15907=CARTESIAN_POINT('Ctrl Pts',(-0.139836317888042,-0.203463743702801,
-0.971100730005489));
#15908=CARTESIAN_POINT('Ctrl Pts',(-0.15681442133453,-0.190326085855194,
-0.968453058988463));
#15909=CARTESIAN_POINT('Ctrl Pts',(-0.1868781821531,-0.15976606450048,-0.963103647174702));
#15910=CARTESIAN_POINT('Ctrl Pts',(-0.199966927975188,-0.142345102874864,
-0.960411259488514));
#15911=CARTESIAN_POINT('Ctrl Pts',(-0.223801617934945,-0.099930567888331,
-0.955173119738174));
#15912=CARTESIAN_POINT('Ctrl Pts',(-0.233157223576062,-0.0740444353928835,
-0.952850216871763));
#15913=CARTESIAN_POINT('Ctrl Pts',(-0.238183666596899,-0.0476299999999999,
-0.951592097314));
#15914=CARTESIAN_POINT('Origin',(5.55111512312578E-17,-0.04763,-1.));
#15915=CARTESIAN_POINT('Origin',(0.,-0.04763,0.));
#15916=CARTESIAN_POINT('',(0.504455939115715,-0.04763,-0.841298510752802));
#15917=CARTESIAN_POINT('Origin',(0.,-0.04763,0.));
#15918=CARTESIAN_POINT('Origin',(0.707106781186548,-0.04763,-0.707106781186547));
#15919=CARTESIAN_POINT('Origin',(0.707106781186548,0.,-0.707106781186547));
#15920=CARTESIAN_POINT('',(0.841298510752802,-0.04763,-0.504455939115715));
#15921=CARTESIAN_POINT('Ctrl Pts',(0.841298510752802,-0.04763,-0.504455939115715));
#15922=CARTESIAN_POINT('Ctrl Pts',(0.838633903678357,-0.0740444353928835,
-0.508899795931835));
#15923=CARTESIAN_POINT('Ctrl Pts',(0.833661031856294,-0.0999305678883309,
-0.517157748491652));
#15924=CARTESIAN_POINT('Ctrl Pts',(0.820511285096538,-0.142345102874864,
-0.537715343527944));
#15925=CARTESIAN_POINT('Ctrl Pts',(0.813159949759,-0.159766064500479,-0.548874290046456));
#15926=CARTESIAN_POINT('Ctrl Pts',(0.795684265985088,-0.190326085855194,
-0.573915184558107));
#15927=CARTESIAN_POINT('Ctrl Pts',(0.78555112003688,-0.203463743702801,
-0.587792702767295));
#15928=CARTESIAN_POINT('Ctrl Pts',(0.763642258217233,-0.224161999508995,
-0.615966552324775));
#15929=CARTESIAN_POINT('Ctrl Pts',(0.750785745543687,-0.232861760990032,
-0.631684198665438));
#15930=CARTESIAN_POINT('Ctrl Pts',(0.722929908501543,-0.244251601209411,
-0.663382628119203));
#15931=CARTESIAN_POINT('Ctrl Pts',(0.707917883896095,-0.246942143572133,
-0.679352081686668));
#15932=CARTESIAN_POINT('Ctrl Pts',(0.679352081686668,-0.246942143572133,
-0.707917883896095));
#15933=CARTESIAN_POINT('Ctrl Pts',(0.663382628119203,-0.244251601209411,
-0.722929908501543));
#15934=CARTESIAN_POINT('Ctrl Pts',(0.631684198665438,-0.232861760990032,
-0.750785745543687));
#15935=CARTESIAN_POINT('Ctrl Pts',(0.615966552324775,-0.224161999508995,
-0.763642258217232));
#15936=CARTESIAN_POINT('Ctrl Pts',(0.587792702767295,-0.203463743702801,
-0.78555112003688));
#15937=CARTESIAN_POINT('Ctrl Pts',(0.573915184558107,-0.190326085855194,
-0.795684265985088));
#15938=CARTESIAN_POINT('Ctrl Pts',(0.548874290046456,-0.159766064500479,
-0.813159949759));
#15939=CARTESIAN_POINT('Ctrl Pts',(0.537715343527944,-0.142345102874864,
-0.820511285096538));
#15940=CARTESIAN_POINT('Ctrl Pts',(0.517157748491652,-0.099930567888331,
-0.833661031856294));
#15941=CARTESIAN_POINT('Ctrl Pts',(0.508899795931835,-0.0740444353928835,
-0.838633903678357));
#15942=CARTESIAN_POINT('Ctrl Pts',(0.504455939115715,-0.04763,-0.841298510752801));
#15943=CARTESIAN_POINT('Origin',(0.707106781186548,-0.04763,-0.707106781186547));
#15944=CARTESIAN_POINT('Origin',(0.,-0.166705,0.));
#15945=CARTESIAN_POINT('',(-0.980948,-0.28578,1.20131482833E-16));
#15946=CARTESIAN_POINT('Origin',(0.,-0.28578,0.));
#15947=CARTESIAN_POINT('',(-0.980948,-0.166705,1.20131482833E-16));
#15948=CARTESIAN_POINT('',(0.951592097314,-0.04763,0.238183666596899));
#15949=CARTESIAN_POINT('Origin',(0.,-0.04763,0.));
#15950=CARTESIAN_POINT('',(0.951592097314,-0.04763,-0.238183666596899));
#15951=CARTESIAN_POINT('Ctrl Pts',(0.951592097314,-0.04763,0.238183666596899));
#15952=CARTESIAN_POINT('Ctrl Pts',(0.952850216871763,-0.0740444353928835,
0.233157223576062));
#15953=CARTESIAN_POINT('Ctrl Pts',(0.955173119738174,-0.099930567888331,
0.223801617934945));
#15954=CARTESIAN_POINT('Ctrl Pts',(0.960411259488514,-0.142345102874864,
0.199966927975188));
#15955=CARTESIAN_POINT('Ctrl Pts',(0.963103647174702,-0.15976606450048,
0.1868781821531));
#15956=CARTESIAN_POINT('Ctrl Pts',(0.968453058988463,-0.190326085855194,
0.15681442133453));
#15957=CARTESIAN_POINT('Ctrl Pts',(0.971100730005489,-0.203463743702801,
0.139836317888042));
#15958=CARTESIAN_POINT('Ctrl Pts',(0.975530745318961,-0.224161999508995,
0.104422493053067));
#15959=CARTESIAN_POINT('Ctrl Pts',(0.977553872336861,-0.232861760990032,
0.0842175114474172));
#15960=CARTESIAN_POINT('Ctrl Pts',(0.980270995488453,-0.244251601209411,
0.0421062857595697));
#15961=CARTESIAN_POINT('Ctrl Pts',(0.980948,-0.246942143572133,0.0201990724523194));
#15962=CARTESIAN_POINT('Ctrl Pts',(0.980948,-0.246942143572133,-0.0201990724523194));
#15963=CARTESIAN_POINT('Ctrl Pts',(0.980270995488453,-0.244251601209411,
-0.0421062857595697));
#15964=CARTESIAN_POINT('Ctrl Pts',(0.977553872336861,-0.232861760990032,
-0.0842175114474172));
#15965=CARTESIAN_POINT('Ctrl Pts',(0.975530745318961,-0.224161999508995,
-0.104422493053067));
#15966=CARTESIAN_POINT('Ctrl Pts',(0.971100730005489,-0.203463743702801,
-0.139836317888042));
#15967=CARTESIAN_POINT('Ctrl Pts',(0.968453058988463,-0.190326085855194,
-0.15681442133453));
#15968=CARTESIAN_POINT('Ctrl Pts',(0.963103647174702,-0.15976606450048,
-0.1868781821531));
#15969=CARTESIAN_POINT('Ctrl Pts',(0.960411259488514,-0.142345102874864,
-0.199966927975188));
#15970=CARTESIAN_POINT('Ctrl Pts',(0.955173119738174,-0.099930567888331,
-0.223801617934945));
#15971=CARTESIAN_POINT('Ctrl Pts',(0.952850216871763,-0.0740444353928835,
-0.233157223576062));
#15972=CARTESIAN_POINT('Ctrl Pts',(0.951592097314,-0.0476299999999999,-0.238183666596899));
#15973=CARTESIAN_POINT('Origin',(0.,-0.04763,0.));
#15974=CARTESIAN_POINT('Origin',(0.,-0.04763,0.));
#15975=CARTESIAN_POINT('Origin',(1.,-0.04763,0.));
#15976=CARTESIAN_POINT('Origin',(1.,0.,0.));
#15977=CARTESIAN_POINT('Origin',(1.,-0.04763,0.));
#15978=CARTESIAN_POINT('Origin',(0.,-0.28578,0.));
#15979=CARTESIAN_POINT('Origin',(0.,-0.04763,0.));
#16835=UNCERTAINTY_MEASURE_WITH_UNIT(LENGTH_MEASURE(0.001),#16912,
'DISTANCE_ACCURACY_VALUE',
'Maximum model space distance between geometric entities at asserted c
onnectivities');
#16852=UNCERTAINTY_MEASURE_WITH_UNIT(LENGTH_MEASURE(0.001),#16912,
'DISTANCE_ACCURACY_VALUE',
'Maximum model space distance between geometric entities at asserted c
onnectivities');
#16894=(
GEOMETRIC_REPRESENTATION_CONTEXT(3)
GLOBAL_UNCERTAINTY_ASSIGNED_CONTEXT((#16835))
GLOBAL_UNIT_ASSIGNED_CONTEXT((#16912,#16914,#16915))
REPRESENTATION_CONTEXT('','3D')
);
#16911=(
GEOMETRIC_REPRESENTATION_CONTEXT(3)
GLOBAL_UNCERTAINTY_ASSIGNED_CONTEXT((#16852))
GLOBAL_UNIT_ASSIGNED_CONTEXT((#16912,#16914,#16915))
REPRESENTATION_CONTEXT('','3D')
);
#16912=(
LENGTH_UNIT()
NAMED_UNIT(*)
SI_UNIT(.CENTI.,.METRE.)
);
#16914=(
NAMED_UNIT(*)
PLANE_ANGLE_UNIT()
SI_UNIT($,.RADIAN.)
);
#16915=(
NAMED_UNIT(*)
SI_UNIT($,.STERADIAN.)
SOLID_ANGLE_UNIT()
);
#16957=SHAPE_DEFINITION_REPRESENTATION(#17017,#17165);
#17017=PRODUCT_DEFINITION_SHAPE('',$,#17224);
#17165=SHAPE_REPRESENTATION('',(#10164),#16894);
#17182=PRODUCT_DEFINITION_CONTEXT('part definition',#17358,'design');
#17224=PRODUCT_DEFINITION('Cage','Cage',#17282,#17182);
#17282=PRODUCT_DEFINITION_FORMATION('',$,#17401);
#17358=APPLICATION_CONTEXT(
'Core Data for Automotive Mechanical Design Process');
#17359=PRODUCT_CONTEXT('part definition',#17358,'mechanical');
#17401=PRODUCT('Cage','Cage','Cage',(#17359));
#17481=COLOUR_RGB('Grey',0.48,0.52,0.57);
#17482=FILL_AREA_STYLE_COLOUR('',#17481);
#17483=FILL_AREA_STYLE('',(#17482));
#17484=SURFACE_STYLE_FILL_AREA(#17483);
#17485=SURFACE_SIDE_STYLE('',(#17484));
#17486=SURFACE_STYLE_USAGE(.BOTH.,#17485);
#17487=PRESENTATION_STYLE_ASSIGNMENT((#17486));
ENDSEC;
END-ISO-10303-21;
